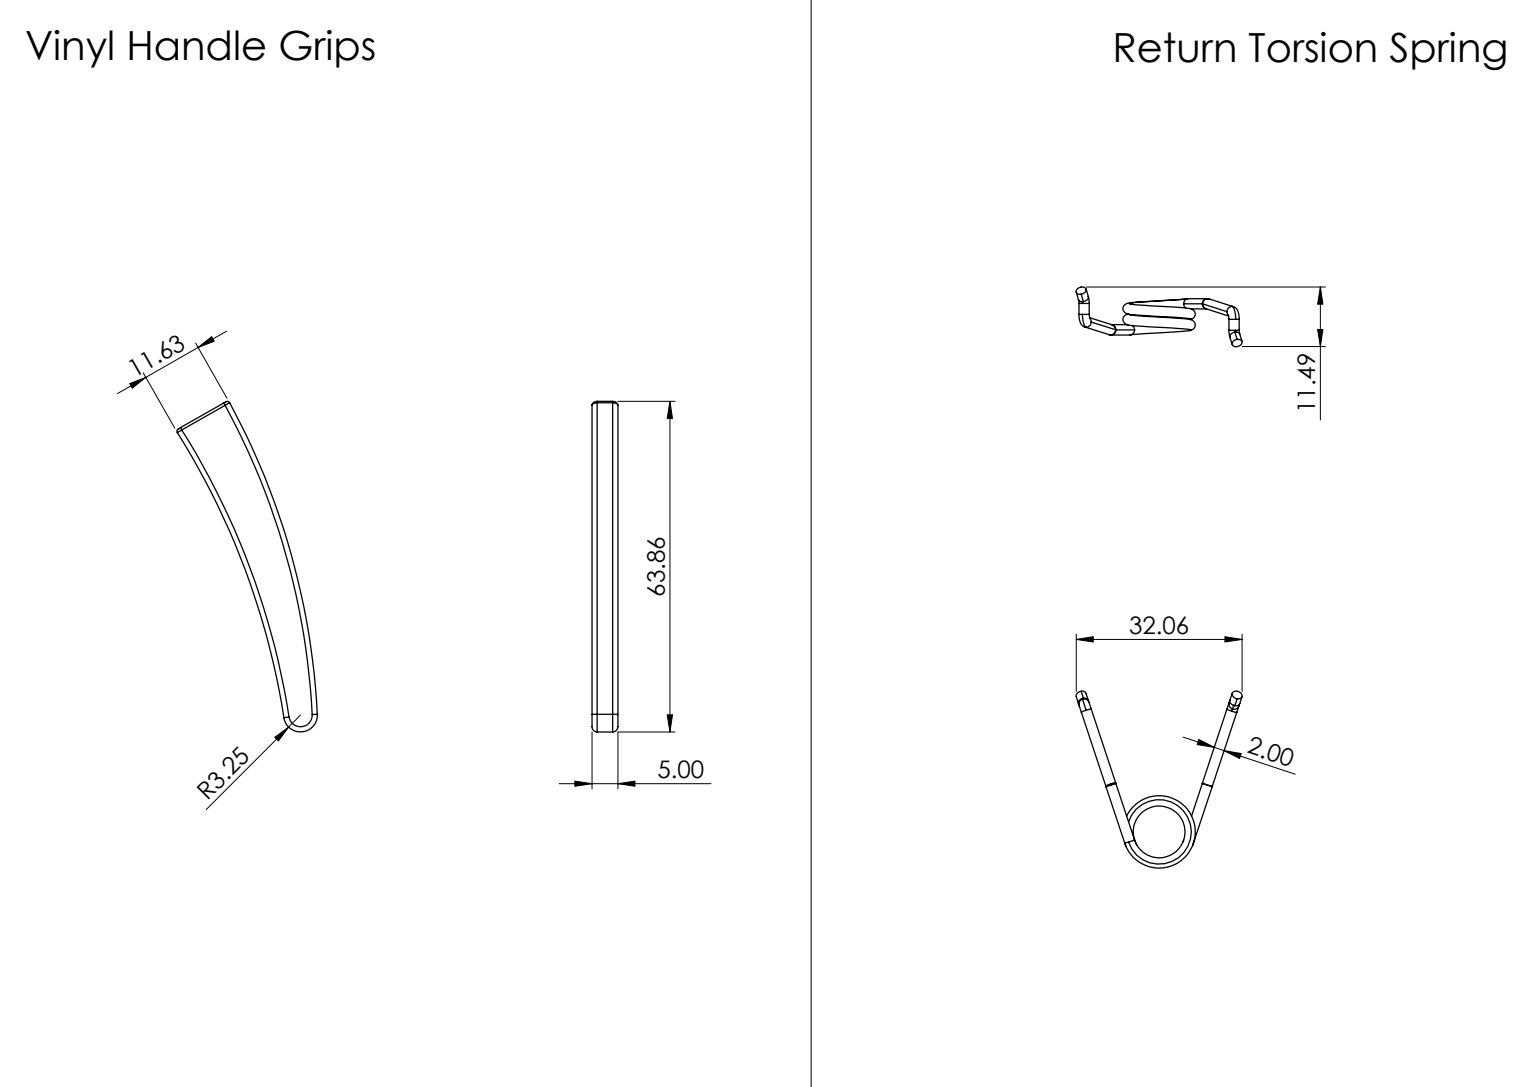
ISO-10303-21;
HEADER;
FILE_DESCRIPTION (('STEP AP214'),
    '1' );
FILE_NAME ('Vinyl Handle Grips.step',
    '2026-10-09T15:01:35',
    ( '' ),
    ( '' ),
    'SwSTEP 2.0',
    'SolidWorks 2026',
    '' );
FILE_SCHEMA (( 'AUTOMOTIVE_DESIGN' ));
ENDSEC;

DATA;
#1=ORIENTED_EDGE ( 'NONE', *, *, #451, .F. ) ;
#30=CARTESIAN_POINT ( 'NONE',  ( 27.63595919327375938, -34.25856858997740062, -0.5081525913518375459 ) ) ;
#33=ORIENTED_EDGE ( 'NONE', *, *, #2628, .F. ) ;
#46=ORIENTED_EDGE ( 'NONE', *, *, #4272, .T. ) ;
#49=DIRECTION ( 'NONE',  ( 5.715354789845005112E-18, 9.999836672264339449E-16, -1.000000000000000000 ) ) ;
#51=SURFACE_STYLE_USAGE ( .BOTH. , #5819 ) ;
#52=DIRECTION ( 'NONE',  ( 0.000000000000000000, -1.000000000000000000, -9.973300763855647239E-16 ) ) ;
#60=CARTESIAN_POINT ( 'NONE',  ( 17.88843813672053074, -40.41242482140540204, -4.025211077939831437E-14 ) ) ;
#61=DIRECTION ( 'NONE',  ( -0.9999836672264333925, 0.005715354789844476896, 0.000000000000000000 ) ) ;
#69=CARTESIAN_POINT ( 'NONE',  ( 18.49916120972752154, -39.46430250869199341, 3.499999999999960476 ) ) ;
#72=CARTESIAN_POINT ( 'NONE',  ( 26.87031364676133194, -34.69479876584122024, -0.5000000000000345279 ) ) ;
#83=LINE ( 'NONE', #2969, #2404 ) ;
#84=EDGE_CURVE ( 'NONE', #5434, #6822, #3844, .T. ) ;
#91=CARTESIAN_POINT ( 'NONE',  ( 18.31438873653245381, -40.15745658308031807, 3.873766277856072193 ) ) ;
#93=FACE_OUTER_BOUND ( 'NONE', #5404, .T. ) ;
#107=CARTESIAN_POINT ( 'NONE',  ( 27.99155020439382469, -34.64269665048638558, -3.446982116472166490E-14 ) ) ;
#131=ORIENTED_EDGE ( 'NONE', *, *, #84, .F. ) ;
#136=CARTESIAN_POINT ( 'NONE',  ( 27.99155020439386377, -34.64269665048637137, -4.257530847521587323E-14 ) ) ;
#140=EDGE_CURVE ( 'NONE', #6822, #6113, #1025, .T. ) ;
#166=DIRECTION ( 'NONE',  ( 5.715354789845005112E-18, 9.999836672264339449E-16, -1.000000000000000000 ) ) ;
#169=CIRCLE ( 'NONE', #2691, 147.0000000000000000 ) ;
#183=ORIENTED_EDGE ( 'NONE', *, *, #2628, .T. ) ;
#185=( LENGTH_UNIT ( ) NAMED_UNIT ( * ) SI_UNIT ( .MILLI., .METRE. ) );
#202=CYLINDRICAL_SURFACE ( 'NONE', #2445, 0.5000000000000022204 ) ;
#227=DIRECTION ( 'NONE',  ( 5.715354789845004342E-18, 9.999836672264337477E-16, -1.000000000000000000 ) ) ;
#234=TOROIDAL_SURFACE ( 'NONE', #5408, 140.0000000000000000, 1.000000000000000000 ) ;
#235=EDGE_CURVE ( 'NONE', #5505, #4310, #421, .T. ) ;
#237=CARTESIAN_POINT ( 'NONE',  ( 18.49916120972751088, -39.46430250869199341, -0.5000000000000393019 ) ) ;
#245=CARTESIAN_POINT ( 'NONE',  ( -105.7473861751082040, -118.0666774205683822, 2.999999999999881428 ) ) ;
#253=EDGE_CURVE ( 'NONE', #4908, #2830, #5444, .T. ) ;
#261=EDGE_CURVE ( 'NONE', #1236, #2830, #5625, .T. ) ;
#274=UNCERTAINTY_MEASURE_WITH_UNIT (LENGTH_MEASURE( 1.000000000000000082E-05 ), #185, 'distance_accuracy_value', 'NONE');
#275=AXIS2_PLACEMENT_3D ( 'NONE', #245, #7168, #3592 ) ;
#294=ORIENTED_EDGE ( 'NONE', *, *, #1501, .T. ) ;
#298=CIRCLE ( 'NONE', #3775, 145.9999999999999716 ) ;
#313=CARTESIAN_POINT ( 'NONE',  ( 27.55235279947361349, -34.88166451341158592, 3.999999999999965361 ) ) ;
#318=CARTESIAN_POINT ( 'NONE',  ( -95.86211798318534250, -102.0316339954322018, 3.999999999999897859 ) ) ;
#344=CARTESIAN_POINT ( 'NONE',  ( 18.49916120972752509, -39.46430250869199341, 3.499999999999960476 ) ) ;
#349=FACE_OUTER_BOUND ( 'NONE', #6871, .T. ) ;
#360=FACE_OUTER_BOUND ( 'NONE', #2389, .T. ) ;
#368=DIRECTION ( 'NONE',  ( 5.715354789845005112E-18, 9.999836672264339449E-16, -1.000000000000000000 ) ) ;
#370=DIRECTION ( 'NONE',  ( -0.9999836672264335036, 0.005715354789845008589, 0.000000000000000000 ) ) ;
#372=ORIENTED_EDGE ( 'NONE', *, *, #5459, .F. ) ;
#375=CARTESIAN_POINT ( 'NONE',  ( 39.48483786921892857, -95.33781693134928048, 3.999999999999904521 ) ) ;
#386=CARTESIAN_POINT ( 'NONE',  ( -105.7473861751082040, -118.0666774205683822, 2.999999999999881428 ) ) ;
#387=CARTESIAN_POINT ( 'NONE',  ( -95.86211798318534250, -102.0316339954322018, 2.999999999999897859 ) ) ;
#391=AXIS2_PLACEMENT_3D ( 'NONE', #5186, #5641, #2797 ) ;
#393=EDGE_CURVE ( 'NONE', #1414, #6322, #2060, .T. ) ;
#401=CARTESIAN_POINT ( 'NONE',  ( 27.74785680215192940, -34.19481439742430240, 3.132117371547133100 ) ) ;
#403=ORIENTED_EDGE ( 'NONE', *, *, #803, .T. ) ;
#407=AXIS2_PLACEMENT_3D ( 'NONE', #1418, #3070, #5386 ) ;
#420=VERTEX_POINT ( 'NONE', #6767 ) ;
#421=LINE ( 'NONE', #2456, #6291 ) ;
#445=EDGE_LOOP ( 'NONE', ( #6799, #6289, #2155, #183 ) ) ;
#446=ORIENTED_EDGE ( 'NONE', *, *, #1818, .F. ) ;
#450=CARTESIAN_POINT ( 'NONE',  ( 41.70778007397900211, -94.98992620957551480, 2.999999999999905409 ) ) ;
#451=EDGE_CURVE ( 'NONE', #5505, #7068, #7351, .T. ) ;
#453=LINE ( 'NONE', #485, #6901 ) ;
#456=CARTESIAN_POINT ( 'NONE',  ( -109.1076725891878567, -112.1689003517234227, -1.127570259384924611E-13 ) ) ;
#460=ORIENTED_EDGE ( 'NONE', *, *, #4272, .F. ) ;
#462=CARTESIAN_POINT ( 'NONE',  ( 18.23198843067283548, -39.61652546476334180, 3.399839610809888946 ) ) ;
#463=DIRECTION ( 'NONE',  ( 0.9986925448795958005, 0.05111947575940636868, 0.000000000000000000 ) ) ;
#466=CARTESIAN_POINT ( 'NONE',  ( 27.55235279947335414, -34.88166451341171381, -3.471129529363089628E-14 ) ) ;
#471=CARTESIAN_POINT ( 'NONE',  ( 18.47982041150265431, -39.47532202006953383, -3.946495907847236140E-14 ) ) ;
#474=CARTESIAN_POINT ( 'NONE',  ( 18.06432739836633061, -39.71205113188396041, -3.955074325938771262E-14 ) ) ;
#481=CARTESIAN_POINT ( 'NONE',  ( -105.7473861751082040, -118.0666774205683822, -1.186117176699141851E-13 ) ) ;
#485=CARTESIAN_POINT ( 'NONE',  ( 18.06432739836633061, -39.71205113188396041, 3.999999999999960032 ) ) ;
#502=CARTESIAN_POINT ( 'NONE',  ( 18.74668230531433721, -39.89873697698325117, 3.999999999999960032 ) ) ;
#515=CARTESIAN_POINT ( 'NONE',  ( 18.38437304540687833, -39.52970360889655410, -0.5000000000000393019 ) ) ;
#527=AXIS2_PLACEMENT_3D ( 'NONE', #7403, #2247, #4554 ) ;
#530=DIRECTION ( 'NONE',  ( 0.000000000000000000, -1.000000000000000000, -8.673617379884027583E-16 ) ) ;
#531=DIRECTION ( 'NONE',  ( -0.9999836672264333925, 0.005715354789843017994, -1.984263399433601008E-30 ) ) ;
#533=LINE ( 'NONE', #2887, #6913 ) ;
#546=ORIENTED_EDGE ( 'NONE', *, *, #3188, .T. ) ;
#555=VERTEX_POINT ( 'NONE', #5918 ) ;
#556=B_SPLINE_CURVE_WITH_KNOTS ( 'NONE', 3,
 ( #5245, #2849, #6332, #5736, #1652, #5167, #596, #5949 ),
 .UNSPECIFIED., .F., .F.,
 ( 4, 2, 2, 4 ),
 ( 7.023086426956682172E-18, 0.0003905485738067056029, 0.0007810971476134041585, 0.001562194295226800728 ),
 .UNSPECIFIED. ) ;
#584=CARTESIAN_POINT ( 'NONE',  ( 18.49916120972750377, -39.46430250869199341, -0.5000000000000393019 ) ) ;
#592=CARTESIAN_POINT ( 'NONE',  ( 27.24990648202821575, -34.47852395037432416, -0.2518834531394323339 ) ) ;
#596=CARTESIAN_POINT ( 'NONE',  ( 27.99155020439387798, -34.64269665048637137, -0.2641155699549361247 ) ) ;
#612=CARTESIAN_POINT ( 'NONE',  ( 17.98171507014359349, -40.35658427893240230, 3.523056311642938088 ) ) ;
#618=CARTESIAN_POINT ( 'NONE',  ( 27.57050386326208979, -34.29586207421746735, 3.619543086858307390 ) ) ;
#626=CARTESIAN_POINT ( 'NONE',  ( 18.11162751801429849, -39.68510166472335499, 3.261603458983328263 ) ) ;
#631=CARTESIAN_POINT ( 'NONE',  ( 27.88111011609792556, -34.70420074580282943, -0.5037669066447876265 ) ) ;
#637=TOROIDAL_SURFACE ( 'NONE', #2433, 2.249999999999964917, 1.000000000000000000 ) ;
#647=AXIS2_PLACEMENT_3D ( 'NONE', #7275, #6601, #6098 ) ;
#673=CARTESIAN_POINT ( 'NONE',  ( 18.06432739836606771, -39.71205113188410962, 2.999999999999960476 ) ) ;
#676=EDGE_CURVE ( 'NONE', #888, #2009, #2043, .T. ) ;
#706=ADVANCED_FACE ( 'NONE', ( #360 ), #1383, .T. ) ;
#709=AXIS2_PLACEMENT_3D ( 'NONE', #6443, #2440, #1841 ) ;
#717=DIRECTION ( 'NONE',  ( 5.715354789845005112E-18, 9.999836672264339449E-16, -1.000000000000000000 ) ) ;
#718=CARTESIAN_POINT ( 'NONE',  ( 39.48483786921892857, -95.33781693134928048, 3.999999999999904521 ) ) ;
#721=CARTESIAN_POINT ( 'NONE',  ( 18.11927033577788393, -39.68074713310974744, -0.2519513543403087419 ) ) ;
#731=CARTESIAN_POINT ( 'NONE',  ( 26.87807528571524074, -34.69037653529182563, 2.999999999999965361 ) ) ;
#745=CIRCLE ( 'NONE', #1355, 147.0000000000000000 ) ;
#750=EDGE_CURVE ( 'NONE', #6928, #6113, #6639, .T. ) ;
#751=AXIS2_PLACEMENT_3D ( 'NONE', #5959, #3597, #6467 ) ;
#762=CARTESIAN_POINT ( 'NONE',  ( -95.86211798318534250, -102.0316339954322018, 3.999999999999897859 ) ) ;
#763=CARTESIAN_POINT ( 'NONE',  ( 17.88843813772660596, -40.41242482300715011, -0.1308508315819079393 ) ) ;
#765=CIRCLE ( 'NONE', #6539, 0.5000000000000004441 ) ;
#767=AXIS2_PLACEMENT_3D ( 'NONE', #871, #3769, #5908 ) ;
#774=AXIS2_PLACEMENT_3D ( 'NONE', #1957, #4270, #4224 ) ;
#802=EDGE_CURVE ( 'NONE', #7250, #6854, #6673, .T. ) ;
#803=EDGE_CURVE ( 'NONE', #5496, #7250, #1244, .T. ) ;
#816=DIRECTION ( 'NONE',  ( -5.715354789845005112E-18, -9.999836672264339449E-16, 1.000000000000000000 ) ) ;
#818=CARTESIAN_POINT ( 'NONE',  ( 27.11783474234813340, -35.12923323413248511, 3.499999999999964917 ) ) ;
#819=DIRECTION ( 'NONE',  ( -0.9999836672264335036, 0.005715354789845008589, 0.000000000000000000 ) ) ;
#824=CYLINDRICAL_SURFACE ( 'NONE', #5814, 2.249999999999962252 ) ;
#851=ORIENTED_EDGE ( 'NONE', *, *, #4724, .T. ) ;
#863=STYLED_ITEM ( 'NONE', ( #5858 ), #2394 ) ;
#869=TOROIDAL_SURFACE ( 'NONE', #275, 147.0000000000000000, 1.000000000000000000 ) ;
#871=CARTESIAN_POINT ( 'NONE',  ( 27.55235279947361349, -34.88166451341158592, 3.999999999999965361 ) ) ;
#884=CARTESIAN_POINT ( 'NONE',  ( 17.88843813672055916, -40.41242482140537362, 3.999999999999959144 ) ) ;
#888=VERTEX_POINT ( 'NONE', #5085 ) ;
#896=DIRECTION ( 'NONE',  ( 5.715354789845005112E-18, 9.999836672264339449E-16, -1.000000000000000000 ) ) ;
#911=FACE_OUTER_BOUND ( 'NONE', #4195, .T. ) ;
#927=ORIENTED_EDGE ( 'NONE', *, *, #5460, .F. ) ;
#932=DIRECTION ( 'NONE',  ( 5.715354789845005112E-18, 9.999836672264339449E-16, -1.000000000000000000 ) ) ;
#936=VERTEX_POINT ( 'NONE', #107 ) ;
#939=LINE ( 'NONE', #456, #5214 ) ;
#941=DIRECTION ( 'NONE',  ( 5.715354789845005112E-18, 9.999836672264339449E-16, -1.000000000000000000 ) ) ;
#958=CARTESIAN_POINT ( 'NONE',  ( 27.99155020439384955, -34.64269665048638558, 2.999999999999965361 ) ) ;
#968=FACE_OUTER_BOUND ( 'NONE', #3719, .T. ) ;
#989=( GEOMETRIC_REPRESENTATION_CONTEXT ( 3 ) GLOBAL_UNCERTAINTY_ASSIGNED_CONTEXT ( ( #274 ) ) GLOBAL_UNIT_ASSIGNED_CONTEXT ( ( #185, #5991, #3638 ) ) REPRESENTATION_CONTEXT ( 'NONE', 'WORKASPACE' ) );
#1002=ORIENTED_EDGE ( 'NONE', *, *, #7088, .T. ) ;
#1004=ORIENTED_EDGE ( 'NONE', *, *, #7088, .F. ) ;
#1006=CIRCLE ( 'NONE', #647, 147.0000000000000000 ) ;
#1014=EDGE_LOOP ( 'NONE', ( #403, #1276, #2986, #6808 ) ) ;
#1021=CARTESIAN_POINT ( 'NONE',  ( 27.88123484459569568, -34.70413128614676168, 3.503735202131379900 ) ) ;
#1024=ORIENTED_EDGE ( 'NONE', *, *, #261, .T. ) ;
#1025=B_SPLINE_CURVE_WITH_KNOTS ( 'NONE', 3,
 ( #4575, #3398, #2302, #91, #1665, #612, #4005, #4077 ),
 .UNSPECIFIED., .F., .F.,
 ( 4, 2, 2, 4 ),
 ( 0.000000000000000000, 0.0003905813100143790020, 0.0007811626200287574619, 0.001562325240057513189 ),
 .UNSPECIFIED. ) ;
#1027=CARTESIAN_POINT ( 'NONE',  ( 17.79267347262679522, -39.86682724249966014, 3.626282107859409187 ) ) ;
#1032=DIRECTION ( 'NONE',  ( -3.391455187862681927E-16, -1.191495097990696953E-15, 1.000000000000000000 ) ) ;
#1055=DIRECTION ( 'NONE',  ( -3.391455187862681927E-16, -1.191495097990696953E-15, 1.000000000000000000 ) ) ;
#1059=CARTESIAN_POINT ( 'NONE',  ( 27.81639631407590585, -34.74023945865230445, 3.614623298852130517 ) ) ;
#1063=CARTESIAN_POINT ( 'NONE',  ( 18.31450325791856315, -40.15738803827605352, 3.873838653338203208 ) ) ;
#1074=TOROIDAL_SURFACE ( 'NONE', #2746, 140.0000000000000000, 1.000000000000000000 ) ;
#1081=AXIS2_PLACEMENT_3D ( 'NONE', #1259, #3654, #5970 ) ;
#1087=DIRECTION ( 'NONE',  ( 5.715354789845005112E-18, 9.999836672264339449E-16, -1.000000000000000000 ) ) ;
#1092=FACE_OUTER_BOUND ( 'NONE', #2421, .T. ) ;
#1097=CARTESIAN_POINT ( 'NONE',  ( -108.8601514936008385, -112.6033348200152773, 3.499999999999886757 ) ) ;
#1098=DIRECTION ( 'NONE',  ( -5.715354789845005112E-18, -9.999836672264339449E-16, 1.000000000000000000 ) ) ;
#1101=ORIENTED_EDGE ( 'NONE', *, *, #3974, .T. ) ;
#1117=ORIENTED_EDGE ( 'NONE', *, *, #1901, .T. ) ;
#1123=AXIS2_PLACEMENT_3D ( 'NONE', #4973, #5514, #2057 ) ;
#1131=EDGE_LOOP ( 'NONE', ( #4538, #294, #3018, #5684 ) ) ;
#1140=VECTOR ( 'NONE', #4420, 1000.000000000000000 ) ;
#1142=LINE ( 'NONE', #2372, #5672 ) ;
#1159=DIRECTION ( 'NONE',  ( -2.925622616928933849E-16, -1.164954066665946421E-15, 1.000000000000000000 ) ) ;
#1166=CYLINDRICAL_SURFACE ( 'NONE', #527, 0.5000000000000004441 ) ;
#1168=CARTESIAN_POINT ( 'NONE',  ( 27.55792021817859805, -34.88417811465595264, -0.8737629652053834350 ) ) ;
#1177=CARTESIAN_POINT ( 'NONE',  ( -105.7473861751082040, -118.0666774205683822, 3.999999999999881428 ) ) ;
#1181=CARTESIAN_POINT ( 'NONE',  ( 18.44231076305980466, -39.49669331989797172, 3.499999956044343552 ) ) ;
#1182=EDGE_CURVE ( 'NONE', #6822, #2064, #5580, .T. ) ;
#1189=DIRECTION ( 'NONE',  ( -0.9879743132267160277, -0.1546180985661085583, 0.000000000000000000 ) ) ;
#1197=ORIENTED_EDGE ( 'NONE', *, *, #7043, .T. ) ;
#1198=VERTEX_POINT ( 'NONE', #6993 ) ;
#1203=FACE_OUTER_BOUND ( 'NONE', #5268, .T. ) ;
#1231=VERTEX_POINT ( 'NONE', #2096 ) ;
#1236=VERTEX_POINT ( 'NONE', #2622 ) ;
#1244=CIRCLE ( 'NONE', #391, 0.5000000000000022204 ) ;
#1259=CARTESIAN_POINT ( 'NONE',  ( -95.86211798318534250, -102.0316339954322018, 2.999999999999897859 ) ) ;
#1264=APPLICATION_CONTEXT ( 'automotive_design' ) ;
#1268=CARTESIAN_POINT ( 'NONE',  ( 17.99687608643026593, -40.34751144403527690, -0.5039026972369210489 ) ) ;
#1276=ORIENTED_EDGE ( 'NONE', *, *, #3188, .F. ) ;
#1283=CARTESIAN_POINT ( 'NONE',  ( 27.30483170388658110, -34.44723004512043474, -3.833102624698575208E-14 ) ) ;
#1297=DIRECTION ( 'NONE',  ( -0.4950421911735689018, 0.8688689365825386091, 0.000000000000000000 ) ) ;
#1306=ORIENTED_EDGE ( 'NONE', *, *, #4864, .T. ) ;
#1309=DIRECTION ( 'NONE',  ( -0.9999836672264335036, 0.005715354789845041548, 0.000000000000000000 ) ) ;
#1312=ORIENTED_EDGE ( 'NONE', *, *, #7327, .F. ) ;
#1316=DIRECTION ( 'NONE',  ( -0.9879743132267160277, -0.1546180985661085583, -1.602621969470663276E-16 ) ) ;
#1321=ADVANCED_FACE ( 'NONE', ( #5573 ), #6181, .T. ) ;
#1332=CARTESIAN_POINT ( 'NONE',  ( 18.06432743677800445, -39.71205110999872545, -0.06542542002766411902 ) ) ;
#1354=VERTEX_POINT ( 'NONE', #2703 ) ;
#1355=AXIS2_PLACEMENT_3D ( 'NONE', #1984, #816, #5967 ) ;
#1359=SURFACE_STYLE_FILL_AREA ( #4219 ) ;
#1370=DIRECTION ( 'NONE',  ( -0.9999836672264333925, 0.005715354789844984303, 0.000000000000000000 ) ) ;
#1379=CIRCLE ( 'NONE', #7379, 1.000000000000001998 ) ;
#1383=( BOUNDED_SURFACE ( )  B_SPLINE_SURFACE ( 3, 2, ( 
 ( #4396, #6133, #958 ),
 ( #5566, #401, #2694 ),
 ( #3894, #5069, #5115 ),
 ( #4013, #6208, #6828 ),
 ( #7352, #618, #7395 ),
 ( #6352, #6867, #1713 ),
 ( #3477, #4546, #5152 ),
 ( #1756, #4052, #7313 ),
 ( #6278, #4512, #5676 ),
 ( #3928, #4627, #6318 ) ),
 .UNSPECIFIED., .F., .F., .F. ) 
 B_SPLINE_SURFACE_WITH_KNOTS ( ( 4, 2, 2, 2, 4 ),
 ( 3, 3 ),
 ( -2.981555974335137194E-18, 0.0001952886961233724105, 0.0003905773922467478025, 0.0005858660883701231675, 0.0007811547844934985324 ),
 ( 0.000000000000000000, 1.000000000000000000 ),
 .UNSPECIFIED. ) 
 GEOMETRIC_REPRESENTATION_ITEM ( )  RATIONAL_B_SPLINE_SURFACE ( (
 ( 1.000000000000000000, 0.7001503461741274137, 1.000000000000000000),
 ( 1.000000000000000000, 0.7001491056773789801, 1.000000000000000000),
 ( 1.000000000000000000, 0.7003313827919757095, 1.000000000000000000),
 ( 1.000000000000000000, 0.7010298770397929147, 1.000000000000000000),
 ( 1.000000000000000000, 0.7015467090662059757, 1.000000000000000000),
 ( 1.000000000000000000, 0.7028299121717020981, 1.000000000000000000),
 ( 1.000000000000000000, 0.7036054228162287316, 1.000000000000000000),
 ( 1.000000000000000000, 0.7052774926288423174, 1.000000000000000000),
 ( 1.000000000000000000, 0.7061929979163744653, 1.000000000000000000),
 ( 1.000000000000000000, 0.7071067811865477948, 1.000000000000000000) ) ) 
 REPRESENTATION_ITEM ( '' )  SURFACE ( )  );
#1408=ORIENTED_EDGE ( 'NONE', *, *, #7380, .T. ) ;
#1414=VERTEX_POINT ( 'NONE', #6324 ) ;
#1418=CARTESIAN_POINT ( 'NONE',  ( -105.7473861751082040, -118.0666774205683822, 3.999999999999881428 ) ) ;
#1430=LINE ( 'NONE', #3720, #3512 ) ;
#1443=DIRECTION ( 'NONE',  ( 5.715354789845005112E-18, 9.999836672264339449E-16, -1.000000000000000000 ) ) ;
#1478=AXIS2_PLACEMENT_3D ( 'NONE', #481, #368, #6653 ) ;
#1488=AXIS2_PLACEMENT_3D ( 'NONE', #3820, #1087, #370 ) ;
#1501=EDGE_CURVE ( 'NONE', #6491, #1414, #1839, .T. ) ;
#1534=FACE_OUTER_BOUND ( 'NONE', #5497, .T. ) ;
#1535=DIRECTION ( 'NONE',  ( 5.715354789845005112E-18, 9.999836672264339449E-16, -1.000000000000000000 ) ) ;
#1539=EDGE_CURVE ( 'NONE', #6928, #1231, #5117, .T. ) ;
#1549=DIRECTION ( 'NONE',  ( -5.715354789845005112E-18, -9.999836672264339449E-16, 1.000000000000000000 ) ) ;
#1565=ORIENTED_EDGE ( 'NONE', *, *, #253, .T. ) ;
#1596=ORIENTED_EDGE ( 'NONE', *, *, #3604, .F. ) ;
#1604=LINE ( 'NONE', #884, #4615 ) ;
#1625=CARTESIAN_POINT ( 'NONE',  ( 18.38544986348231447, -39.52909008669877977, 3.487024505045074996 ) ) ;
#1629=CARTESIAN_POINT ( 'NONE',  ( 18.74668230531428748, -39.89873697698326538, -1.000000000000039968 ) ) ;
#1652=CARTESIAN_POINT ( 'NONE',  ( 27.65482637540493016, -34.83021424519443343, -0.7995430095508657686 ) ) ;
#1655=CARTESIAN_POINT ( 'NONE',  ( 27.57479190627129384, -34.87478370679277617, 3.891341692651370199 ) ) ;
#1665=CARTESIAN_POINT ( 'NONE',  ( 18.21922820888615036, -40.21441497322944514, 3.799573870912058116 ) ) ;
#1681=ADVANCED_FACE ( 'NONE', ( #7059 ), #2390, .F. ) ;
#1700=CARTESIAN_POINT ( 'NONE',  ( 18.06097555607235705, -40.30914097186184364, 3.615364355270606289 ) ) ;
#1705=ORIENTED_EDGE ( 'NONE', *, *, #5741, .T. ) ;
#1713=CARTESIAN_POINT ( 'NONE',  ( 27.65530182349729671, -34.82994948188742512, 3.799124122364484712 ) ) ;
#1720=VECTOR ( 'NONE', #6644, 1000.000000000000000 ) ;
#1721=PRODUCT_CONTEXT ( 'NONE', #1264, 'mechanical' ) ;
#1727=CARTESIAN_POINT ( 'NONE',  ( 27.11783474234811564, -35.12923323413249221, -1.000000000000034861 ) ) ;
#1744=AXIS2_PLACEMENT_3D ( 'NONE', #762, #1916, #4877 ) ;
#1756=CARTESIAN_POINT ( 'NONE',  ( 26.98470030103655404, -34.62962642788639300, 3.486735179637458604 ) ) ;
#1768=ORIENTED_EDGE ( 'NONE', *, *, #393, .F. ) ;
#1778=DIRECTION ( 'NONE',  ( 5.715354789845004342E-18, 9.999836672264337477E-16, -1.000000000000000000 ) ) ;
#1779=CARTESIAN_POINT ( 'NONE',  ( 43.95483829995806957, -94.87490738911687060, 2.999999999999905409 ) ) ;
#1786=DIRECTION ( 'NONE',  ( -0.1546180985661130547, 0.9879743132267154726, 9.870744795757317374E-16 ) ) ;
#1798=CARTESIAN_POINT ( 'NONE',  ( 27.65480120734329006, -34.83022826066387267, -0.7995651912284664764 ) ) ;
#1803=ADVANCED_BREP_SHAPE_REPRESENTATION ( '', ( #2394, #751 ), #989 ) ;
#1816=ORIENTED_EDGE ( 'NONE', *, *, #3604, .T. ) ;
#1818=EDGE_CURVE ( 'NONE', #2009, #6491, #1006, .T. ) ;
#1824=ORIENTED_EDGE ( 'NONE', *, *, #5459, .T. ) ;
#1839=CIRCLE ( 'NONE', #4008, 2.249999999999962252 ) ;
#1841=DIRECTION ( 'NONE',  ( -0.9999836672264332815, 0.005715354789842956411, 0.000000000000000000 ) ) ;
#1844=AXIS2_PLACEMENT_3D ( 'NONE', #2492, #166, #1370 ) ;
#1847=AXIS2_PLACEMENT_3D ( 'NONE', #7148, #227, #2518 ) ;
#1854=ORIENTED_EDGE ( 'NONE', *, *, #6843, .F. ) ;
#1885=CYLINDRICAL_SURFACE ( 'NONE', #2212, 0.5000000000000004441 ) ;
#1886=CARTESIAN_POINT ( 'NONE',  ( 17.61082888335783991, -39.97043405836763696, -0.1337947118489001552 ) ) ;
#1901=EDGE_CURVE ( 'NONE', #3586, #5496, #6981, .T. ) ;
#1916=DIRECTION ( 'NONE',  ( -5.715354789845005112E-18, -9.999836672264339449E-16, 1.000000000000000000 ) ) ;
#1917=FACE_OUTER_BOUND ( 'NONE', #3479, .T. ) ;
#1957=CARTESIAN_POINT ( 'NONE',  ( 41.70778007397900211, -94.98992620957551480, -1.000000000000094591 ) ) ;
#1958=CARTESIAN_POINT ( 'NONE',  ( 18.74668230531429458, -39.89873697698326538, -1.000000000000039746 ) ) ;
#1984=CARTESIAN_POINT ( 'NONE',  ( -105.7473861751082040, -118.0666774205683822, -1.000000000000118794 ) ) ;
#2009=VERTEX_POINT ( 'NONE', #471 ) ;
#2016=ORIENTED_EDGE ( 'NONE', *, *, #1182, .T. ) ;
#2034=ORIENTED_EDGE ( 'NONE', *, *, #802, .F. ) ;
#2036=EDGE_CURVE ( 'NONE', #420, #7068, #3939, .T. ) ;
#2043=LINE ( 'NONE', #4352, #1720 ) ;
#2048=ORIENTED_EDGE ( 'NONE', *, *, #3336, .T. ) ;
#2057=DIRECTION ( 'NONE',  ( -0.9999836672264333925, 0.005715354789844970425, 0.000000000000000000 ) ) ;
#2060=CIRCLE ( 'NONE', #5815, 140.0000000000000000 ) ;
#2064=VERTEX_POINT ( 'NONE', #718 ) ;
#2068=CARTESIAN_POINT ( 'NONE',  ( 41.70778007397900211, -94.98992620957551480, 3.999999999999905409 ) ) ;
#2086=ADVANCED_FACE ( 'NONE', ( #3800 ), #7117, .T. ) ;
#2087=ADVANCED_FACE ( 'NONE', ( #911 ), #824, .F. ) ;
#2091=ORIENTED_EDGE ( 'NONE', *, *, #5846, .F. ) ;
#2096=CARTESIAN_POINT ( 'NONE',  ( 18.49916120972752154, -39.46430250869199341, 3.499999999999960476 ) ) ;
#2100=EDGE_LOOP ( 'NONE', ( #446, #5456, #4019, #5209 ) ) ;
#2107=DIRECTION ( 'NONE',  ( -0.8688689365825387201, -0.4950421911735688463, -4.999999999999992500E-16 ) ) ;
#2150=APPLICATION_CONTEXT ( 'automotive_design' ) ;
#2155=ORIENTED_EDGE ( 'NONE', *, *, #4864, .F. ) ;
#2167=EDGE_CURVE ( 'NONE', #3782, #1414, #1430, .T. ) ;
#2177=AXIS2_PLACEMENT_3D ( 'NONE', #6222, #1055, #530 ) ;
#2184=CIRCLE ( 'NONE', #5086, 2.249999999999962252 ) ;
#2194=ADVANCED_FACE ( 'NONE', ( #3198 ), #4514, .T. ) ;
#2203=EDGE_LOOP ( 'NONE', ( #1705, #5259, #2016, #2577 ) ) ;
#2212=AXIS2_PLACEMENT_3D ( 'NONE', #313, #6561, #6592 ) ;
#2220=CARTESIAN_POINT ( 'NONE',  ( -95.86211798318534250, -102.0316339954322018, -1.025655255171287195E-13 ) ) ;
#2226=CARTESIAN_POINT ( 'NONE',  ( 18.06432739836606771, -39.71205113188410962, 2.999999999999959144 ) ) ;
#2228=CARTESIAN_POINT ( 'NONE',  ( 27.55235279947361349, -34.38166451341171381, -3.421263025543810879E-14 ) ) ;
#2237=LINE ( 'NONE', #4510, #2564 ) ;
#2243=VERTEX_POINT ( 'NONE', #5629 ) ;
#2246=ORIENTED_EDGE ( 'NONE', *, *, #6154, .F. ) ;
#2247=DIRECTION ( 'NONE',  ( 5.715354789845005112E-18, 9.999836672264339449E-16, -1.000000000000000000 ) ) ;
#2249=PLANE ( 'NONE',  #2332 ) ;
#2251=ORIENTED_EDGE ( 'NONE', *, *, #7295, .T. ) ;
#2252=ORIENTED_EDGE ( 'NONE', *, *, #3180, .F. ) ;
#2268=CARTESIAN_POINT ( 'NONE',  ( 18.74668230531428748, -39.89873697698326538, -1.000000000000039968 ) ) ;
#2276=VERTEX_POINT ( 'NONE', #3390 ) ;
#2283=CARTESIAN_POINT ( 'NONE',  ( 27.23210503485723777, -35.06560599256804522, -1.000000000000034861 ) ) ;
#2302=CARTESIAN_POINT ( 'NONE',  ( 18.52216156081266618, -40.03310245541522505, 3.974029017541355291 ) ) ;
#2304=CARTESIAN_POINT ( 'NONE',  ( 39.48483786921892857, -95.33781693134928048, 2.999999999999904521 ) ) ;
#2326=CARTESIAN_POINT ( 'NONE',  ( 27.29329919813223526, -34.45380074488651445, -0.1316498810018032206 ) ) ;
#2332=AXIS2_PLACEMENT_3D ( 'NONE', #5040, #3221, #1535 ) ;
#2346=( LENGTH_UNIT ( ) NAMED_UNIT ( * ) SI_UNIT ( .MILLI., .METRE. ) );
#2357=ADVANCED_FACE ( 'NONE', ( #3499 ), #6967, .T. ) ;
#2363=CARTESIAN_POINT ( 'NONE',  ( 27.96836146114586441, -34.65561064741672226, -0.2632997616376124284 ) ) ;
#2372=CARTESIAN_POINT ( 'NONE',  ( 44.95353084483765826, -94.82378791335750634, 3.999999999999905409 ) ) ;
#2377=( NAMED_UNIT ( * ) SI_UNIT ( $, .STERADIAN. ) SOLID_ANGLE_UNIT ( ) );
#2382=CARTESIAN_POINT ( 'NONE',  ( 18.05682957847944436, -39.71632305027067389, -0.8833408112552532110 ) ) ;
#2386=( BOUNDED_SURFACE ( )  B_SPLINE_SURFACE ( 3, 2, ( 
 ( #2978, #6422, #3055 ),
 ( #1332, #1886, #763 ),
 ( #3661, #5262, #5977 ),
 ( #721, #5935, #1268 ),
 ( #4798, #6482, #4834 ),
 ( #4725, #4160, #3549 ),
 ( #6452, #2382, #3581 ),
 ( #5864, #7081, #3617 ),
 ( #3689, #5896, #5398 ),
 ( #237, #7119, #1958 ) ),
 .UNSPECIFIED., .F., .F., .T. ) 
 B_SPLINE_SURFACE_WITH_KNOTS ( ( 4, 2, 2, 2, 4 ),
 ( 3, 3 ),
 ( 0.000000000000000000, 0.0001953595625521471020, 0.0003907191251042942039, 0.0005860786876564413059, 0.0007814382502085884079 ),
 ( 0.000000000000000000, 1.000000000000000000 ),
 .UNSPECIFIED. ) 
 GEOMETRIC_REPRESENTATION_ITEM ( )  RATIONAL_B_SPLINE_SURFACE ( (
 ( 1.000000000000000000, 0.6917656125192643835, 1.000000000000000000),
 ( 1.000000000000000000, 0.6917626678221141523, 1.000000000000000000),
 ( 1.000000000000000000, 0.6921708295056779869, 1.000000000000000000),
 ( 1.000000000000000000, 0.6937291441607075226, 1.000000000000000000),
 ( 1.000000000000000000, 0.6948807116037144516, 1.000000000000000000),
 ( 1.000000000000000000, 0.6977261400977853301, 1.000000000000000000),
 ( 1.000000000000000000, 0.6994400533938299747, 1.000000000000000000),
 ( 1.000000000000000000, 0.7031153542365370379, 1.000000000000000000),
 ( 1.000000000000000000, 0.7051186676678535825, 1.000000000000000000),
 ( 1.000000000000000000, 0.7071067811865472397, 1.000000000000000000) ) ) 
 REPRESENTATION_ITEM ( '' )  SURFACE ( )  );
#2388=VERTEX_POINT ( 'NONE', #5888 ) ;
#2389=EDGE_LOOP ( 'NONE', ( #3062, #6776, #1824, #6331, #3971 ) ) ;
#2390=PLANE ( 'NONE',  #4114 ) ;
#2393=CARTESIAN_POINT ( 'NONE',  ( 27.57011700825883693, -34.29608248668765214, -0.6201149797898980465 ) ) ;
#2394=MANIFOLD_SOLID_BREP ( 'Stock-MAS-689-1', #3615 ) ;
#2404=VECTOR ( 'NONE', #1098, 1000.000000000000000 ) ;
#2421=EDGE_LOOP ( 'NONE', ( #4697, #4071, #2541, #3463 ) ) ;
#2433=AXIS2_PLACEMENT_3D ( 'NONE', #4645, #7410, #531 ) ;
#2440=DIRECTION ( 'NONE',  ( 5.715354789845005112E-18, 9.999836672264339449E-16, -1.000000000000000000 ) ) ;
#2445=AXIS2_PLACEMENT_3D ( 'NONE', #5326, #2529, #1297 ) ;
#2448=CIRCLE ( 'NONE', #1488, 140.0000000000000000 ) ;
#2455=EDGE_CURVE ( 'NONE', #1198, #3782, #2184, .T. ) ;
#2456=CARTESIAN_POINT ( 'NONE',  ( 27.55235279947361349, -34.38166451341158592, 3.999999999999966249 ) ) ;
#2457=CARTESIAN_POINT ( 'NONE',  ( 18.31184849395284786, -40.14648560017537449, -3.998375596128007773E-14 ) ) ;
#2466=EDGE_CURVE ( 'NONE', #420, #5434, #6057, .T. ) ;
#2467=ORIENTED_EDGE ( 'NONE', *, *, #6733, .F. ) ;
#2492=CARTESIAN_POINT ( 'NONE',  ( -105.7473861751082040, -118.0666774205683822, 3.999999999999881428 ) ) ;
#2518=DIRECTION ( 'NONE',  ( -0.005715354789845003385, -0.9999836672264335036, -1.000000000000000472E-15 ) ) ;
#2526=CARTESIAN_POINT ( 'NONE',  ( 27.09727426766168534, -34.56548687730422387, -0.4458683620789745672 ) ) ;
#2529=DIRECTION ( 'NONE',  ( 0.8688689365825387201, 0.4950421911735688463, 4.999999999999993486E-16 ) ) ;
#2541=ORIENTED_EDGE ( 'NONE', *, *, #6003, .F. ) ;
#2550=DIRECTION ( 'NONE',  ( -5.715354789845005112E-18, -9.999836672264339449E-16, 1.000000000000000000 ) ) ;
#2553=MECHANICAL_DESIGN_GEOMETRIC_PRESENTATION_REPRESENTATION('',(#863),#3627);
#2564=VECTOR ( 'NONE', #6276, 1000.000000000000000 ) ;
#2574=CIRCLE ( 'NONE', #774, 2.249999999999962252 ) ;
#2576=DIRECTION ( 'NONE',  ( -0.9999836672264333925, 0.005715354789844970425, 0.000000000000000000 ) ) ;
#2577=ORIENTED_EDGE ( 'NONE', *, *, #3180, .T. ) ;
#2601=DIRECTION ( 'NONE',  ( -0.005715354789845003385, -0.9999836672264335036, -1.000000000000000472E-15 ) ) ;
#2604=PRODUCT_DEFINITION_CONTEXT ( 'detailed design', #2150, 'design' ) ;
#2610=ORIENTED_EDGE ( 'NONE', *, *, #2167, .F. ) ;
#2622=CARTESIAN_POINT ( 'NONE',  ( 27.30483170388656333, -34.44723004512044895, -3.427979277949995323E-14 ) ) ;
#2626=ORIENTED_EDGE ( 'NONE', *, *, #5743, .T. ) ;
#2628=EDGE_CURVE ( 'NONE', #2388, #4165, #5455, .T. ) ;
#2631=EDGE_LOOP ( 'NONE', ( #5850, #1408, #5648, #7101 ) ) ;
#2635=ADVANCED_FACE ( 'NONE', ( #7437 ), #1166, .T. ) ;
#2637=DIRECTION ( 'NONE',  ( -0.9999836672264333925, 0.005715354789844476896, 0.000000000000000000 ) ) ;
#2663=LINE ( 'NONE', #3374, #4610 ) ;
#2670=AXIS2_PLACEMENT_3D ( 'NONE', #5581, #4301, #4157 ) ;
#2678=UNCERTAINTY_MEASURE_WITH_UNIT (LENGTH_MEASURE( 1.000000000000000082E-05 ), #2346, 'distance_accuracy_value', 'NONE');
#2684=CARTESIAN_POINT ( 'NONE',  ( 27.55235279947333993, -34.88166451341173513, 2.999999999999965361 ) ) ;
#2691=AXIS2_PLACEMENT_3D ( 'NONE', #6675, #4775, #1309 ) ;
#2694=CARTESIAN_POINT ( 'NONE',  ( 27.99155020480830913, -34.64269665124812292, 3.130807245034128883 ) ) ;
#2703=CARTESIAN_POINT ( 'NONE',  ( 39.48483786921892857, -95.33781693134928048, -1.000000000000095035 ) ) ;
#2714=CARTESIAN_POINT ( 'NONE',  ( 18.74668230531430879, -39.89873697698326538, 3.499999999999960032 ) ) ;
#2733=DIRECTION ( 'NONE',  ( -5.715354789845005112E-18, -9.999836672264339449E-16, 1.000000000000000000 ) ) ;
#2741=EDGE_LOOP ( 'NONE', ( #2048, #131, #5871, #2091 ) ) ;
#2742=CARTESIAN_POINT ( 'NONE',  ( 17.91123389404125277, -40.39877837690324469, 3.263394571671051292 ) ) ;
#2746=AXIS2_PLACEMENT_3D ( 'NONE', #6413, #5317, #3544 ) ;
#2754=CARTESIAN_POINT ( 'NONE',  ( 18.27182554301009532, -39.59382808135931242, -0.4457246814534224222 ) ) ;
#2777=ADVANCED_FACE ( 'NONE', ( #4740 ), #869, .T. ) ;
#2793=VECTOR ( 'NONE', #5451, 1000.000000000000000 ) ;
#2797=DIRECTION ( 'NONE',  ( -0.4950421911735689018, 0.8688689365825386091, 0.000000000000000000 ) ) ;
#2802=ORIENTED_EDGE ( 'NONE', *, *, #6003, .T. ) ;
#2804=DIRECTION ( 'NONE',  ( -0.9999836672264333925, 0.005715354789844476896, 0.000000000000000000 ) ) ;
#2811=AXIS2_PLACEMENT_3D ( 'NONE', #4289, #5993, #6141 ) ;
#2818=EDGE_CURVE ( 'NONE', #2276, #6322, #5906, .T. ) ;
#2830=VERTEX_POINT ( 'NONE', #5951 ) ;
#2841=DIRECTION ( 'NONE',  ( -5.715354789845005112E-18, -9.999836672264339449E-16, 1.000000000000000000 ) ) ;
#2847=EDGE_LOOP ( 'NONE', ( #5275, #4432, #6575, #2467 ) ) ;
#2849=CARTESIAN_POINT ( 'NONE',  ( 27.23321219009249816, -35.06498951359424865, -1.000000000000034861 ) ) ;
#2866=CARTESIAN_POINT ( 'NONE',  ( 18.52003153382460354, -40.03437257541853711, -1.000000000000039746 ) ) ;
#2877=CARTESIAN_POINT ( 'NONE',  ( 41.70778007397900211, -94.98992620957551480, -9.475926987523308753E-14 ) ) ;
#2887=CARTESIAN_POINT ( 'NONE',  ( 17.61001731287966265, -39.97089645448942719, 3.499999999999960032 ) ) ;
#2889=CARTESIAN_POINT ( 'NONE',  ( 27.34858876736844380, -35.00074627774458946, 3.999999999999965361 ) ) ;
#2891=CARTESIAN_POINT ( 'NONE',  ( -105.7473861751082040, -118.0666774205683822, 2.999999999999881428 ) ) ;
#2905=EDGE_CURVE ( 'NONE', #6113, #3586, #1604, .T. ) ;
#2921=CARTESIAN_POINT ( 'NONE',  ( 27.34640600250860487, -35.00195951109004255, -0.9740265123469552533 ) ) ;
#2923=AXIS2_PLACEMENT_3D ( 'NONE', #2714, #7158, #3200 ) ;
#2939=FILL_AREA_STYLE_COLOUR ( '', #7001 ) ;
#2954=EDGE_LOOP ( 'NONE', ( #2251, #851, #4981, #1306 ) ) ;
#2967=DIRECTION ( 'NONE',  ( 0.9986925448795958005, 0.05111947575940636868, 5.682652305653510796E-17 ) ) ;
#2969=CARTESIAN_POINT ( 'NONE',  ( 27.99155020439386732, -34.64269665048638558, 3.999999999999966249 ) ) ;
#2978=CARTESIAN_POINT ( 'NONE',  ( 18.06432739836606416, -39.71205113188410252, -3.955074325938786408E-14 ) ) ;
#2986=ORIENTED_EDGE ( 'NONE', *, *, #253, .F. ) ;
#2989=CARTESIAN_POINT ( 'NONE',  ( 27.08917575328167615, -34.57010104422300145, -0.4368814963732711165 ) ) ;
#3018=ORIENTED_EDGE ( 'NONE', *, *, #393, .T. ) ;
#3051=CARTESIAN_POINT ( 'NONE',  ( 26.98506241315388010, -34.62942011279275079, -0.5000000000000346390 ) ) ;
#3055=CARTESIAN_POINT ( 'NONE',  ( 17.88843813672055916, -40.41242482140538073, -4.025211077939830175E-14 ) ) ;
#3062=ORIENTED_EDGE ( 'NONE', *, *, #2466, .T. ) ;
#3070=DIRECTION ( 'NONE',  ( 5.715354789845005112E-18, 9.999836672264339449E-16, -1.000000000000000000 ) ) ;
#3110=PLANE ( 'NONE',  #1847 ) ;
#3113=DIRECTION ( 'NONE',  ( 0.8688689365825388311, 0.4950421911735690128, -8.411011176753756085E-16 ) ) ;
#3119=DIRECTION ( 'NONE',  ( 5.715354789845004342E-18, 9.999836672264337477E-16, -1.000000000000000000 ) ) ;
#3128=AXIS2_PLACEMENT_3D ( 'NONE', #318, #7233, #2576 ) ;
#3129=PRODUCT_DEFINITION_SHAPE ( 'NONE', 'NONE',  #4117 ) ;
#3135=ORIENTED_EDGE ( 'NONE', *, *, #2818, .T. ) ;
#3137=ORIENTED_EDGE ( 'NONE', *, *, #235, .F. ) ;
#3160=AXIS2_PLACEMENT_3D ( 'NONE', #6265, #6342, #52 ) ;
#3170=ORIENTED_EDGE ( 'NONE', *, *, #2455, .T. ) ;
#3178=ORIENTED_EDGE ( 'NONE', *, *, #6154, .T. ) ;
#3180=EDGE_CURVE ( 'NONE', #2064, #7211, #7015, .T. ) ;
#3188=EDGE_CURVE ( 'NONE', #2830, #7250, #2237, .T. ) ;
#3198=FACE_OUTER_BOUND ( 'NONE', #3269, .T. ) ;
#3200=DIRECTION ( 'NONE',  ( -0.4950421911735689018, 0.8688689365825386091, 0.000000000000000000 ) ) ;
#3208=ORIENTED_EDGE ( 'NONE', *, *, #4353, .F. ) ;
#3221=DIRECTION ( 'NONE',  ( 0.4950421911735688463, -0.8688689365825387201, -8.660254037844397269E-16 ) ) ;
#3223=ORIENTED_EDGE ( 'NONE', *, *, #2455, .F. ) ;
#3236=ADVANCED_FACE ( 'NONE', ( #4225 ), #202, .T. ) ;
#3251=ORIENTED_EDGE ( 'NONE', *, *, #2818, .F. ) ;
#3252=ORIENTED_EDGE ( 'NONE', *, *, #5690, .F. ) ;
#3269=EDGE_LOOP ( 'NONE', ( #6616, #6172, #4347, #7146 ) ) ;
#3283=ADVANCED_FACE ( 'NONE', ( #93 ), #6522, .F. ) ;
#3284=ADVANCED_FACE ( 'NONE', ( #1917 ), #2386, .T. ) ;
#3327=CARTESIAN_POINT ( 'NONE',  ( 18.06432739836605350, -39.71205113188411673, -0.1321155921049125825 ) ) ;
#3334=DIRECTION ( 'NONE',  ( -0.4950421911735689018, 0.8688689365825386091, 0.000000000000000000 ) ) ;
#3336=EDGE_CURVE ( 'NONE', #1231, #6822, #4974, .T. ) ;
#3348=FACE_OUTER_BOUND ( 'NONE', #2631, .T. ) ;
#3371=DIRECTION ( 'NONE',  ( 5.715354789845005112E-18, 9.999836672264339449E-16, -1.000000000000000000 ) ) ;
#3374=CARTESIAN_POINT ( 'NONE',  ( 27.30483170388682623, -34.44723004512029974, -3.426145681764390930E-14 ) ) ;
#3388=AXIS2_PLACEMENT_3D ( 'NONE', #818, #3113, #3334 ) ;
#3390=CARTESIAN_POINT ( 'NONE',  ( 26.87807528571524074, -34.69037653529182563, 2.999999999999965361 ) ) ;
#3398=CARTESIAN_POINT ( 'NONE',  ( 18.63335487545880653, -39.96655599946684845, 3.999999999999960032 ) ) ;
#3406=CARTESIAN_POINT ( 'NONE',  ( 18.31184849395311787, -40.14648560017523238, 2.999999999999960032 ) ) ;
#3420=CIRCLE ( 'NONE', #1744, 140.0000000000000000 ) ;
#3430=CARTESIAN_POINT ( 'NONE',  ( 17.99698676687863852, -40.34744519239936267, 3.503909830570486328 ) ) ;
#3452=CARTESIAN_POINT ( 'NONE',  ( 27.13735696382475027, -34.54264957135247016, -0.3997825902234797835 ) ) ;
#3463=ORIENTED_EDGE ( 'NONE', *, *, #5743, .F. ) ;
#3464=CARTESIAN_POINT ( 'NONE',  ( 18.52223854178785345, -40.03305638412986411, 3.974049037550727803 ) ) ;
#3469=ORIENTED_EDGE ( 'NONE', *, *, #7135, .T. ) ;
#3477=CARTESIAN_POINT ( 'NONE',  ( 27.08917652808902687, -34.57010060277283969, 3.436818098114547748 ) ) ;
#3479=EDGE_LOOP ( 'NONE', ( #3931, #5729, #3252, #2034 ) ) ;
#3485=CARTESIAN_POINT ( 'NONE',  ( 27.40755238667390614, -34.38870444966534734, -0.8044411694303389426 ) ) ;
#3499=FACE_OUTER_BOUND ( 'NONE', #5471, .T. ) ;
#3504=EDGE_CURVE ( 'NONE', #936, #4310, #5830, .T. ) ;
#3511=CARTESIAN_POINT ( 'NONE',  ( 41.70778007397900211, -94.98992620957551480, 3.999999999999905409 ) ) ;
#3512=VECTOR ( 'NONE', #6155, 1000.000000000000000 ) ;
#3544=DIRECTION ( 'NONE',  ( -0.9999836672264333925, 0.005715354789844971292, -3.141587852546554631E-32 ) ) ;
#3549=CARTESIAN_POINT ( 'NONE',  ( 18.21884925479887940, -40.21464179917847304, -0.7992328572925022634 ) ) ;
#3562=CARTESIAN_POINT ( 'NONE',  ( 27.74785688037308518, -34.19481435285785409, -4.220975948576798359E-14 ) ) ;
#3581=CARTESIAN_POINT ( 'NONE',  ( 18.31450470689560461, -40.15738718825951992, -0.8737133221916458803 ) ) ;
#3586=VERTEX_POINT ( 'NONE', #5778 ) ;
#3592=DIRECTION ( 'NONE',  ( -0.9999836672264333925, 0.005715354789845005987, 4.554564057672517313E-33 ) ) ;
#3594=DIRECTION ( 'NONE',  ( -5.715354789845005112E-18, -9.999836672264339449E-16, 1.000000000000000000 ) ) ;
#3597=DIRECTION ( 'NONE',  ( 0.000000000000000000, 0.000000000000000000, 1.000000000000000000 ) ) ;
#3604=EDGE_CURVE ( 'NONE', #2388, #7211, #5953, .T. ) ;
#3615=CLOSED_SHELL ( 'NONE', ( #5776, #2777, #6140, #3640, #1321, #7424, #3899, #1681, #2357, #3792, #2087, #3944, #2086, #7095, #5267, #4112, #3283, #6741, #3284, #2635, #3236, #2194, #6936, #4030, #7000, #706 ) ) ;
#3617=CARTESIAN_POINT ( 'NONE',  ( 18.52082317230821928, -40.03390347989001441, -0.9734914404586040293 ) ) ;
#3627=( GEOMETRIC_REPRESENTATION_CONTEXT ( 3 ) GLOBAL_UNCERTAINTY_ASSIGNED_CONTEXT ( ( #2678 ) ) GLOBAL_UNIT_ASSIGNED_CONTEXT ( ( #2346, #4654, #2377 ) ) REPRESENTATION_CONTEXT ( 'NONE', 'WORKASPACE' ) );
#3628=AXIS2_PLACEMENT_3D ( 'NONE', #3406, #1159, #6916 ) ;
#3638=( NAMED_UNIT ( * ) SI_UNIT ( $, .STERADIAN. ) SOLID_ANGLE_UNIT ( ) );
#3640=ADVANCED_FACE ( 'NONE', ( #4107 ), #1074, .T. ) ;
#3652=EDGE_CURVE ( 'NONE', #6398, #2388, #6721, .T. ) ;
#3654=DIRECTION ( 'NONE',  ( 5.715354789845005112E-18, 9.999836672264339449E-16, -1.000000000000000000 ) ) ;
#3661=CARTESIAN_POINT ( 'NONE',  ( 18.07563673267965854, -39.70560758510323041, -0.1308779909158750421 ) ) ;
#3675=CARTESIAN_POINT ( 'NONE',  ( -105.7473861751082040, -118.0666774205683822, -1.186117176699141851E-13 ) ) ;
#3689=CARTESIAN_POINT ( 'NONE',  ( 18.44199058758350063, -39.49687574139178992, -0.4999999711863141738 ) ) ;
#3713=CARTESIAN_POINT ( 'NONE',  ( 43.95483829995806957, -94.87490738911687060, 3.999999999999905409 ) ) ;
#3719=EDGE_LOOP ( 'NONE', ( #5944, #4813, #4631, #1024, #546, #6420, #7201, #6153 ) ) ;
#3720=CARTESIAN_POINT ( 'NONE',  ( 43.95483829995806957, -94.87490738911687060, 3.999999999999905409 ) ) ;
#3725=CARTESIAN_POINT ( 'NONE',  ( 38.49686355599224896, -95.49243502991532750, 2.999999999999904521 ) ) ;
#3736=VECTOR ( 'NONE', #6161, 1000.000000000000000 ) ;
#3754=AXIS2_PLACEMENT_3D ( 'NONE', #6247, #3371, #5124 ) ;
#3757=ORIENTED_EDGE ( 'NONE', *, *, #6221, .F. ) ;
#3759=CARTESIAN_POINT ( 'NONE',  ( 43.95483829995806957, -94.87490738911687060, 2.999999999999905409 ) ) ;
#3769=DIRECTION ( 'NONE',  ( 5.715354789845005112E-18, 9.999836672264339449E-16, -1.000000000000000000 ) ) ;
#3775=AXIS2_PLACEMENT_3D ( 'NONE', #3675, #896, #6545 ) ;
#3782=VERTEX_POINT ( 'NONE', #3759 ) ;
#3792=ADVANCED_FACE ( 'NONE', ( #4262 ), #3829, .F. ) ;
#3800=FACE_OUTER_BOUND ( 'NONE', #6044, .T. ) ;
#3814=EDGE_LOOP ( 'NONE', ( #5910, #1101, #6448, #1596 ) ) ;
#3820=CARTESIAN_POINT ( 'NONE',  ( -95.86211798318534250, -102.0316339954322018, -1.000000000000102807 ) ) ;
#3825=CARTESIAN_POINT ( 'NONE',  ( 27.25760507213267658, -34.47413764220541310, -0.2615252949604586208 ) ) ;
#3829=CYLINDRICAL_SURFACE ( 'NONE', #6138, 140.0000000000000000 ) ;
#3842=DIRECTION ( 'NONE',  ( -7.159176919053500386E-18, -9.973300763855708376E-16, 1.000000000000000000 ) ) ;
#3844=LINE ( 'NONE', #5024, #3736 ) ;
#3863=DIRECTION ( 'NONE',  ( -0.9999836672264335036, 0.005715354789845008589, 0.000000000000000000 ) ) ;
#3868=CYLINDRICAL_SURFACE ( 'NONE', #4936, 0.4999999999999978906 ) ;
#3876=CARTESIAN_POINT ( 'NONE',  ( 17.61082880304171994, -39.97043410412675968, 2.999999999999957812 ) ) ;
#3883=DIRECTION ( 'NONE',  ( 0.000000000000000000, -1.000000000000000000, -8.673617379884027583E-16 ) ) ;
#3894=CARTESIAN_POINT ( 'NONE',  ( 27.29354050645795482, -34.45366325832522136, 3.130828461196526469 ) ) ;
#3899=ADVANCED_FACE ( 'NONE', ( #3348 ), #234, .T. ) ;
#3904=FACE_BOUND ( 'NONE', #4666, .T. ) ;
#3910=ORIENTED_EDGE ( 'NONE', *, *, #4724, .F. ) ;
#3912=( BOUNDED_SURFACE ( )  B_SPLINE_SURFACE ( 3, 2, ( 
 ( #72, #5764, #1727 ),
 ( #5163, #4026, #2283 ),
 ( #4134, #4672, #2921 ),
 ( #2989, #4703, #1168 ),
 ( #3452, #3485, #1798 ),
 ( #5273, #2393, #5804 ),
 ( #592, #30, #631 ),
 ( #2326, #5240, #2363 ),
 ( #6954, #7031, #6435 ),
 ( #1283, #3562, #136 ) ),
 .UNSPECIFIED., .F., .F., .T. ) 
 B_SPLINE_SURFACE_WITH_KNOTS ( ( 4, 2, 2, 2, 4 ),
 ( 3, 3 ),
 ( 0.000000000000000000, 0.0001952887240141836802, 0.0003905774480283673604, 0.0005858661720425509863, 0.0007811548960567347207 ),
 ( 0.000000000000000000, 1.000000000000000000 ),
 .UNSPECIFIED. ) 
 GEOMETRIC_REPRESENTATION_ITEM ( )  RATIONAL_B_SPLINE_SURFACE ( (
 ( 1.000000000000000000, 0.7071067811865472397, 1.000000000000000000),
 ( 1.000000000000000000, 0.7061982418737673406, 1.000000000000000000),
 ( 1.000000000000000000, 0.7052889306346207254, 1.000000000000000000),
 ( 1.000000000000000000, 0.7036054371094994098, 1.000000000000000000),
 ( 1.000000000000000000, 0.7028338995551517421, 1.000000000000000000),
 ( 1.000000000000000000, 0.7015497601672633365, 1.000000000000000000),
 ( 1.000000000000000000, 0.7010307650890416076, 1.000000000000000000),
 ( 1.000000000000000000, 0.7003352509067762854, 1.000000000000000000),
 ( 1.000000000000000000, 0.7001488311338350812, 1.000000000000000000),
 ( 1.000000000000000000, 0.7001503461741274137, 1.000000000000000000) ) ) 
 REPRESENTATION_ITEM ( '' )  SURFACE ( )  );
#3917=CARTESIAN_POINT ( 'NONE',  ( 17.88843813672056626, -40.41242482140539494, 2.999999999999957367 ) ) ;
#3928=CARTESIAN_POINT ( 'NONE',  ( 26.87031364676134970, -34.69479876584121314, 3.499999999999965805 ) ) ;
#3931=ORIENTED_EDGE ( 'NONE', *, *, #803, .F. ) ;
#3939=B_SPLINE_CURVE_WITH_KNOTS ( 'NONE', 3,
 ( #5751, #4832, #5863, #4691, #4158, #5368 ),
 .UNSPECIFIED., .F., .F.,
 ( 4, 2, 4 ),
 ( 0.000000000000000000, 0.0003937726336352555625, 0.0007875452672705111250 ),
 .UNSPECIFIED. ) ;
#3944=ADVANCED_FACE ( 'NONE', ( #6188 ), #4529, .T. ) ;
#3971=ORIENTED_EDGE ( 'NONE', *, *, #2036, .F. ) ;
#3974=EDGE_CURVE ( 'NONE', #6398, #5434, #6402, .T. ) ;
#3990=FACE_OUTER_BOUND ( 'NONE', #2741, .T. ) ;
#3996=CARTESIAN_POINT ( 'NONE',  ( 17.72543015532271937, -39.90513944096638710, 3.513721684389295330 ) ) ;
#4005=CARTESIAN_POINT ( 'NONE',  ( 17.88843813672054850, -40.41242482140538073, 3.264142021185714171 ) ) ;
#4007=AXIS2_PLACEMENT_3D ( 'NONE', #3511, #5225, #61 ) ;
#4008=AXIS2_PLACEMENT_3D ( 'NONE', #2877, #2841, #2804 ) ;
#4013=CARTESIAN_POINT ( 'NONE',  ( 27.24996190780300509, -34.47849237127667266, 3.251881639501436272 ) ) ;
#4019=ORIENTED_EDGE ( 'NONE', *, *, #7011, .T. ) ;
#4020=AXIS2_PLACEMENT_3D ( 'NONE', #387, #3594, #4387 ) ;
#4026=CARTESIAN_POINT ( 'NONE',  ( 26.98408672118752349, -34.62997601791116153, -1.001286369213168825 ) ) ;
#4030=ADVANCED_FACE ( 'NONE', ( #3990 ), #3868, .T. ) ;
#4041=CARTESIAN_POINT ( 'NONE',  ( 18.21934571153571980, -40.21434464133486841, 3.799679232396574236 ) ) ;
#4052=CARTESIAN_POINT ( 'NONE',  ( 27.09963614945447219, -34.56414118396787671, 3.975998075095239503 ) ) ;
#4071=ORIENTED_EDGE ( 'NONE', *, *, #6599, .F. ) ;
#4074=DIRECTION ( 'NONE',  ( 0.05111947575940102573, -0.9986925448795961335, 1.285697817222219874E-14 ) ) ;
#4077=CARTESIAN_POINT ( 'NONE',  ( 17.88843813672055916, -40.41242482140538783, 2.999999999999959588 ) ) ;
#4088=AXIS2_PLACEMENT_3D ( 'NONE', #1177, #5658, #5135 ) ;
#4107=FACE_OUTER_BOUND ( 'NONE', #3814, .T. ) ;
#4112=ADVANCED_FACE ( 'NONE', ( #4649 ), #5964, .T. ) ;
#4114=AXIS2_PLACEMENT_3D ( 'NONE', #6569, #5985, #4843 ) ;
#4117=PRODUCT_DEFINITION ( 'UNKNOWN', '', #6650, #2604 ) ;
#4119=AXIS2_PLACEMENT_3D ( 'NONE', #2891, #1778, #5213 ) ;
#4131=AXIS2_PLACEMENT_3D ( 'NONE', #7217, #2550, #4213 ) ;
#4134=CARTESIAN_POINT ( 'NONE',  ( 26.98398549905668986, -34.63003368969938123, -0.4870132424029344209 ) ) ;
#4157=DIRECTION ( 'NONE',  ( -0.4950421911735689018, 0.8688689365825386091, 0.000000000000000000 ) ) ;
#4158=CARTESIAN_POINT ( 'NONE',  ( 27.30483170388658820, -34.44723004512044184, 3.132067106505118215 ) ) ;
#4160=CARTESIAN_POINT ( 'NONE',  ( 17.95758103425560748, -39.77287037833651340, -0.8100516860784414686 ) ) ;
#4165=VERTEX_POINT ( 'NONE', #3725 ) ;
#4182=ORIENTED_EDGE ( 'NONE', *, *, #6829, .T. ) ;
#4195=EDGE_LOOP ( 'NONE', ( #4553, #4490, #3170, #5481 ) ) ;
#4203=CYLINDRICAL_SURFACE ( 'NONE', #767, 0.5000000000000004441 ) ;
#4213=DIRECTION ( 'NONE',  ( -0.9999836672264332815, 0.005715354789842956411, 0.000000000000000000 ) ) ;
#4219=FILL_AREA_STYLE ('',( #2939 ) ) ;
#4224=DIRECTION ( 'NONE',  ( -0.9999836672264333925, 0.005715354789844476896, 0.000000000000000000 ) ) ;
#4225=FACE_OUTER_BOUND ( 'NONE', #1014, .T. ) ;
#4262=FACE_OUTER_BOUND ( 'NONE', #5768, .T. ) ;
#4267=ORIENTED_EDGE ( 'NONE', *, *, #7135, .F. ) ;
#4270=DIRECTION ( 'NONE',  ( 5.715354789845005112E-18, 9.999836672264339449E-16, -1.000000000000000000 ) ) ;
#4272=EDGE_CURVE ( 'NONE', #4165, #6113, #5782, .T. ) ;
#4289=CARTESIAN_POINT ( 'NONE',  ( 41.70778007397900211, -94.98992620957551480, 2.999999999999905409 ) ) ;
#4301=DIRECTION ( 'NONE',  ( 0.8688689365825388311, 0.4950421911735690128, 0.000000000000000000 ) ) ;
#4304=FACE_OUTER_BOUND ( 'NONE', #6191, .T. ) ;
#4310=VERTEX_POINT ( 'NONE', #2228 ) ;
#4337=DIRECTION ( 'NONE',  ( 5.715354789845005112E-18, 9.999836672264339449E-16, -1.000000000000000000 ) ) ;
#4347=ORIENTED_EDGE ( 'NONE', *, *, #3336, .F. ) ;
#4352=CARTESIAN_POINT ( 'NONE',  ( 18.47982041150265431, -39.47532202006953383, 2.999999999999960476 ) ) ;
#4353=EDGE_CURVE ( 'NONE', #2276, #888, #5556, .T. ) ;
#4358=ORIENTED_EDGE ( 'NONE', *, *, #7011, .F. ) ;
#4379=CIRCLE ( 'NONE', #5472, 0.5000000000000004441 ) ;
#4387=DIRECTION ( 'NONE',  ( -0.9999836672264335036, 0.005715354789845008589, 0.000000000000000000 ) ) ;
#4396=CARTESIAN_POINT ( 'NONE',  ( 27.30483170388657044, -34.44723004512044895, 2.999999999999965805 ) ) ;
#4406=DIRECTION ( 'NONE',  ( -5.715354789845133764E-18, -9.999836672264337477E-16, 1.000000000000000000 ) ) ;
#4420=DIRECTION ( 'NONE',  ( 0.8688689365825387201, 0.4950421911735688463, 4.999999999999993486E-16 ) ) ;
#4432=ORIENTED_EDGE ( 'NONE', *, *, #2905, .F. ) ;
#4452=CARTESIAN_POINT ( 'NONE',  ( 18.05682814888138665, -39.71632386479095089, 3.883467497571597704 ) ) ;
#4482=CARTESIAN_POINT ( 'NONE',  ( -95.86211798318534250, -102.0316339954322018, -1.025655255171287195E-13 ) ) ;
#4490=ORIENTED_EDGE ( 'NONE', *, *, #7227, .F. ) ;
#4496=CARTESIAN_POINT ( 'NONE',  ( 18.11932642638120328, -39.68071517522289327, 3.251954915088070663 ) ) ;
#4510=CARTESIAN_POINT ( 'NONE',  ( 18.47982041150265786, -39.47532202006954094, -0.5000000000000394129 ) ) ;
#4512=CARTESIAN_POINT ( 'NONE',  ( 26.98474422010017904, -34.62960140479226112, 4.001293834245286618 ) ) ;
#4514=( BOUNDED_SURFACE ( )  B_SPLINE_SURFACE ( 3, 2, ( 
 ( #344, #7417, #502 ),
 ( #1181, #6307, #4568 ),
 ( #1625, #7302, #3464 ),
 ( #6902, #4452, #1063 ),
 ( #462, #5098, #4041 ),
 ( #6856, #1027, #1700 ),
 ( #4496, #3996, #3430 ),
 ( #6341, #5056, #2742 ),
 ( #5707, #5742, #5172 ),
 ( #2226, #3876, #3917 ) ),
 .UNSPECIFIED., .F., .F., .F. ) 
 B_SPLINE_SURFACE_WITH_KNOTS ( ( 4, 2, 2, 2, 4 ),
 ( 3, 3 ),
 ( 0.000000000000000000, 0.0001953596913251163321, 0.0003907193826502326642, 0.0005860790739753490505, 0.0007814387653004653284 ),
 ( 0.000000000000000000, 1.000000000000000000 ),
 .UNSPECIFIED. ) 
 GEOMETRIC_REPRESENTATION_ITEM ( )  RATIONAL_B_SPLINE_SURFACE ( (
 ( 1.000000000000000000, 0.7071067811865465735, 1.000000000000000000),
 ( 1.000000000000000000, 0.7051297887126681818, 1.000000000000000000),
 ( 1.000000000000000000, 0.7031405235181358293, 1.000000000000000000),
 ( 1.000000000000000000, 0.6994400710090995510, 1.000000000000000000),
 ( 1.000000000000000000, 0.6977350462886972027, 1.000000000000000000),
 ( 1.000000000000000000, 0.6948874123953024950, 1.000000000000000000),
 ( 1.000000000000000000, 0.6937311395898003719, 1.000000000000000000),
 ( 1.000000000000000000, 0.6921794382103451104, 1.000000000000000000),
 ( 1.000000000000000000, 0.6917621249165484265, 1.000000000000000000),
 ( 1.000000000000000000, 0.6917656125192588323, 1.000000000000000000) ) ) 
 REPRESENTATION_ITEM ( '' )  SURFACE ( )  );
#4529=CYLINDRICAL_SURFACE ( 'NONE', #4088, 147.0000000000000000 ) ;
#4538=ORIENTED_EDGE ( 'NONE', *, *, #1818, .T. ) ;
#4546=CARTESIAN_POINT ( 'NONE',  ( 27.31013720395375799, -34.44420721133294450, 3.877994099121481852 ) ) ;
#4553=ORIENTED_EDGE ( 'NONE', *, *, #1501, .F. ) ;
#4554=DIRECTION ( 'NONE',  ( 0.000000000000000000, 1.000000000000000000, 1.734723475976805517E-15 ) ) ;
#4568=CARTESIAN_POINT ( 'NONE',  ( 18.63446967293817735, -39.96588886641734462, 3.999999999999968026 ) ) ;
#4575=CARTESIAN_POINT ( 'NONE',  ( 18.74668230531430169, -39.89873697698325117, 3.999999999999960032 ) ) ;
#4584=ORIENTED_EDGE ( 'NONE', *, *, #3504, .T. ) ;
#4604=CARTESIAN_POINT ( 'NONE',  ( 27.99155020439383890, -34.64269665048639979, 2.999999999999965805 ) ) ;
#4610=VECTOR ( 'NONE', #6287, 1000.000000000000000 ) ;
#4615=VECTOR ( 'NONE', #1443, 1000.000000000000000 ) ;
#4627=CARTESIAN_POINT ( 'NONE',  ( 26.87031364676134970, -34.69479876584121314, 3.999999999999965361 ) ) ;
#4631=ORIENTED_EDGE ( 'NONE', *, *, #6843, .T. ) ;
#4633=AXIS2_PLACEMENT_3D ( 'NONE', #2457, #7049, #6007 ) ;
#4634=AXIS2_PLACEMENT_3D ( 'NONE', #2304, #1786, #1189 ) ;
#4642=ORIENTED_EDGE ( 'NONE', *, *, #140, .T. ) ;
#4645=CARTESIAN_POINT ( 'NONE',  ( 41.70778007397900211, -94.98992620957551480, -9.475926987523308753E-14 ) ) ;
#4649=FACE_OUTER_BOUND ( 'NONE', #445, .T. ) ;
#4654=( NAMED_UNIT ( * ) PLANE_ANGLE_UNIT ( ) SI_UNIT ( $, .RADIAN. ) );
#4666=EDGE_LOOP ( 'NONE', ( #1312, #3251, #7220, #4822 ) ) ;
#4672=CARTESIAN_POINT ( 'NONE',  ( 27.09819939871877637, -34.56495977950342535, -0.9765397587610813446 ) ) ;
#4681=DIRECTION ( 'NONE',  ( 5.715354789845005112E-18, 9.999836672264339449E-16, -1.000000000000000000 ) ) ;
#4682=ORIENTED_EDGE ( 'NONE', *, *, #235, .T. ) ;
#4691=CARTESIAN_POINT ( 'NONE',  ( 27.25776622504945124, -34.47404582456791644, 3.261208021432587589 ) ) ;
#4697=ORIENTED_EDGE ( 'NONE', *, *, #6506, .T. ) ;
#4699=VECTOR ( 'NONE', #2107, 1000.000000000000000 ) ;
#4703=CARTESIAN_POINT ( 'NONE',  ( 27.31013562793543770, -34.44420810927673671, -0.8781215038714056398 ) ) ;
#4710=CARTESIAN_POINT ( 'NONE',  ( 17.88843813672055916, -40.41242482140538783, 2.999999999999959588 ) ) ;
#4724=EDGE_CURVE ( 'NONE', #936, #6398, #83, .T. ) ;
#4725=CARTESIAN_POINT ( 'NONE',  ( 18.23173688611030485, -39.61666878346903076, -0.3996164340295632611 ) ) ;
#4740=FACE_OUTER_BOUND ( 'NONE', #7139, .T. ) ;
#4758=CARTESIAN_POINT ( 'NONE',  ( 27.30483170388656333, -34.44723004512044895, -0.1320675480243696243 ) ) ;
#4775=DIRECTION ( 'NONE',  ( 5.715354789845005112E-18, 9.999836672264339449E-16, -1.000000000000000000 ) ) ;
#4780=SHAPE_REPRESENTATION_RELATIONSHIP ( 'NONE' , 'NONE' ,  #5284, #1803 ) ;
#4787=CARTESIAN_POINT ( 'NONE',  ( 27.30483170388682979, -34.44723004512030684, 2.999999999999965805 ) ) ;
#4798=CARTESIAN_POINT ( 'NONE',  ( 18.15155958994787611, -39.66235017763963810, -0.3073999163891736330 ) ) ;
#4801=FACE_OUTER_BOUND ( 'NONE', #2954, .T. ) ;
#4813=ORIENTED_EDGE ( 'NONE', *, *, #2036, .T. ) ;
#4822=ORIENTED_EDGE ( 'NONE', *, *, #676, .T. ) ;
#4829=ORIENTED_EDGE ( 'NONE', *, *, #6959, .T. ) ;
#4832=CARTESIAN_POINT ( 'NONE',  ( 26.98506203061672792, -34.62942033074510562, 3.499999999999965361 ) ) ;
#4834=CARTESIAN_POINT ( 'NONE',  ( 18.06060404229330985, -40.30936335904925727, -0.6147998435448814858 ) ) ;
#4843=DIRECTION ( 'NONE',  ( -0.005715354789845003385, -0.9999836672264335036, -1.000000000000000472E-15 ) ) ;
#4856=LINE ( 'NONE', #6693, #7385 ) ;
#4862=CIRCLE ( 'NONE', #4131, 3.250000000000000888 ) ;
#4864=EDGE_CURVE ( 'NONE', #2388, #2243, #1142, .T. ) ;
#4876=CARTESIAN_POINT ( 'NONE',  ( 26.87031364676133194, -34.69479876584122024, -0.5000000000000345279 ) ) ;
#4877=DIRECTION ( 'NONE',  ( -0.9999836672264335036, 0.005715354789845008589, 0.000000000000000000 ) ) ;
#4908=VERTEX_POINT ( 'NONE', #6170 ) ;
#4936=AXIS2_PLACEMENT_3D ( 'NONE', #1097, #7413, #5089 ) ;
#4973=CARTESIAN_POINT ( 'NONE',  ( -95.86211798318534250, -102.0316339954322018, -1.025655255171287195E-13 ) ) ;
#4974=CIRCLE ( 'NONE', #2923, 0.5000000000000022204 ) ;
#4981=ORIENTED_EDGE ( 'NONE', *, *, #3652, .T. ) ;
#4988=LINE ( 'NONE', #5493, #1140 ) ;
#4990=DIRECTION ( 'NONE',  ( 0.000000000000000000, -1.000000000000000000, -9.973300763855647239E-16 ) ) ;
#5012=CARTESIAN_POINT ( 'NONE',  ( 18.49916120972750377, -39.46430250869199341, -0.5000000000000393019 ) ) ;
#5024=CARTESIAN_POINT ( 'NONE',  ( -108.8601514936008385, -112.6033348200152915, 3.999999999999886313 ) ) ;
#5034=ORIENTED_EDGE ( 'NONE', *, *, #6959, .F. ) ;
#5040=CARTESIAN_POINT ( 'NONE',  ( 17.61001731287966265, -39.97089645448942719, 3.999999999999960032 ) ) ;
#5056=CARTESIAN_POINT ( 'NONE',  ( 17.63495400270750224, -39.95668865737157205, 3.269138726291231034 ) ) ;
#5069=CARTESIAN_POINT ( 'NONE',  ( 27.72483002872544944, -34.20793401062830696, 3.264201108005380547 ) ) ;
#5085=CARTESIAN_POINT ( 'NONE',  ( 18.47982041150265431, -39.47532202006953383, 2.999999999999960476 ) ) ;
#5086=AXIS2_PLACEMENT_3D ( 'NONE', #450, #2733, #6554 ) ;
#5089=DIRECTION ( 'NONE',  ( 0.4950421911735801705, -0.8688689365825322808, 0.000000000000000000 ) ) ;
#5098=CARTESIAN_POINT ( 'NONE',  ( 17.95809745115200684, -39.77257614736446811, 3.810493591301452820 ) ) ;
#5104=CARTESIAN_POINT ( 'NONE',  ( 27.55235279947361349, -34.38166451341173513, 2.999999999999965805 ) ) ;
#5115=CARTESIAN_POINT ( 'NONE',  ( 27.96884669319430827, -34.65534042161862516, 3.261656933814885306 ) ) ;
#5117=B_SPLINE_CURVE_WITH_KNOTS ( 'NONE', 3,
 ( #5123, #7435, #626, #5236, #6245, #69 ),
 .UNSPECIFIED., .F., .F.,
 ( 4, 2, 4 ),
 ( 0.000000000000000000, 0.0003939438732545951058, 0.0007878877465091902116 ),
 .UNSPECIFIED. ) ;
#5123=CARTESIAN_POINT ( 'NONE',  ( 18.06432739836606771, -39.71205113188410962, 2.999999999999960476 ) ) ;
#5124=DIRECTION ( 'NONE',  ( -0.9999836672264332815, 0.005715354789842956411, 0.000000000000000000 ) ) ;
#5134=CARTESIAN_POINT ( 'NONE',  ( 38.49686355599224896, -95.49243502991532750, -9.519295074422728931E-14 ) ) ;
#5135=DIRECTION ( 'NONE',  ( -0.9999836672264335036, 0.005715354789845041548, 0.000000000000000000 ) ) ;
#5149=CARTESIAN_POINT ( 'NONE',  ( 17.88843813672053429, -40.41242482140540204, -0.1320686260247052324 ) ) ;
#5152=CARTESIAN_POINT ( 'NONE',  ( 27.55792178321159014, -34.88417723535314252, 3.873636197071128606 ) ) ;
#5163=CARTESIAN_POINT ( 'NONE',  ( 26.92714173160467084, -34.66242069539057979, -0.4999999559301231411 ) ) ;
#5167=CARTESIAN_POINT ( 'NONE',  ( 27.89660656231303193, -34.69557212064219698, -0.5230190109555528100 ) ) ;
#5172=CARTESIAN_POINT ( 'NONE',  ( 17.88843813737523192, -40.41242482244771850, 3.131634423728840488 ) ) ;
#5186=CARTESIAN_POINT ( 'NONE',  ( 18.74668230531428748, -39.89873697698326538, -0.5000000000000397460 ) ) ;
#5203=CARTESIAN_POINT ( 'NONE',  ( 39.48483786921892857, -95.33781693134928048, -9.519295074422728931E-14 ) ) ;
#5209=ORIENTED_EDGE ( 'NONE', *, *, #7227, .T. ) ;
#5213=DIRECTION ( 'NONE',  ( -0.005715354789845003385, -0.9999836672264335036, -1.000000000000000472E-15 ) ) ;
#5214=VECTOR ( 'NONE', #6769, 1000.000000000000000 ) ;
#5225=DIRECTION ( 'NONE',  ( -5.715354789845005112E-18, -9.999836672264339449E-16, 1.000000000000000000 ) ) ;
#5236=CARTESIAN_POINT ( 'NONE',  ( 18.27210872828645094, -39.59366673520705859, 3.445918334850228693 ) ) ;
#5240=CARTESIAN_POINT ( 'NONE',  ( 27.72433805554270592, -34.20821431467933138, -0.2658584296617393372 ) ) ;
#5245=CARTESIAN_POINT ( 'NONE',  ( 27.11783474234811919, -35.12923323413248511, -1.000000000000035083 ) ) ;
#5249=DIRECTION ( 'NONE',  ( 0.05111947575940102573, -0.9986925448795961335, -9.983840675197624659E-16 ) ) ;
#5259=ORIENTED_EDGE ( 'NONE', *, *, #84, .T. ) ;
#5262=CARTESIAN_POINT ( 'NONE',  ( 17.63445134299215056, -39.95697505012468298, -0.2674678461753002279 ) ) ;
#5267=ADVANCED_FACE ( 'NONE', ( #4801 ), #6050, .T. ) ;
#5268=EDGE_LOOP ( 'NONE', ( #1565, #6832, #927, #6738, #5878 ) ) ;
#5273=CARTESIAN_POINT ( 'NONE',  ( 27.21752237596963298, -34.49697494815714549, -0.3076110668159389161 ) ) ;
#5275=ORIENTED_EDGE ( 'NONE', *, *, #5690, .T. ) ;
#5284=SHAPE_REPRESENTATION ( 'Vinyl Handle Grips', ( #751 ), #989 ) ;
#5317=DIRECTION ( 'NONE',  ( 5.715354789845005112E-18, 9.999836672264339449E-16, -1.000000000000000000 ) ) ;
#5326=CARTESIAN_POINT ( 'NONE',  ( 17.85753840846644636, -40.40533092278068494, -0.5000000000000403011 ) ) ;
#5368=CARTESIAN_POINT ( 'NONE',  ( 27.30483170388682979, -34.44723004512030684, 2.999999999999965805 ) ) ;
#5386=DIRECTION ( 'NONE',  ( -0.9999836672264335036, 0.005715354789845041548, 0.000000000000000000 ) ) ;
#5390=FACE_OUTER_BOUND ( 'NONE', #2203, .T. ) ;
#5398=CARTESIAN_POINT ( 'NONE',  ( 18.63383769599579054, -39.96626706310059518, -1.000000000000039746 ) ) ;
#5404=EDGE_LOOP ( 'NONE', ( #46, #7102, #3178, #3757 ) ) ;
#5408=AXIS2_PLACEMENT_3D ( 'NONE', #2220, #49, #5740 ) ;
#5434=VERTEX_POINT ( 'NONE', #6233 ) ;
#5444=CIRCLE ( 'NONE', #2670, 0.5000000000000022204 ) ;
#5445=ORIENTED_EDGE ( 'NONE', *, *, #5460, .T. ) ;
#5451=DIRECTION ( 'NONE',  ( 5.715354789845005112E-18, 9.999836672264339449E-16, -1.000000000000000000 ) ) ;
#5455=CIRCLE ( 'NONE', #3754, 3.250000000000000888 ) ;
#5456=ORIENTED_EDGE ( 'NONE', *, *, #676, .F. ) ;
#5459=EDGE_CURVE ( 'NONE', #6398, #5505, #765, .T. ) ;
#5460=EDGE_CURVE ( 'NONE', #4310, #1236, #4379, .T. ) ;
#5471=EDGE_LOOP ( 'NONE', ( #4358, #3208, #5034, #3223 ) ) ;
#5472=AXIS2_PLACEMENT_3D ( 'NONE', #466, #3842, #4990 ) ;
#5481=ORIENTED_EDGE ( 'NONE', *, *, #2167, .T. ) ;
#5493=CARTESIAN_POINT ( 'NONE',  ( 27.12559638130199247, -35.12481100358304076, -1.000000000000035083 ) ) ;
#5496=VERTEX_POINT ( 'NONE', #1629 ) ;
#5497=EDGE_LOOP ( 'NONE', ( #1816, #2252, #4267, #33 ) ) ;
#5505=VERTEX_POINT ( 'NONE', #5104 ) ;
#5514=DIRECTION ( 'NONE',  ( -5.715354789845005112E-18, -9.999836672264339449E-16, 1.000000000000000000 ) ) ;
#5556=LINE ( 'NONE', #6266, #4699 ) ;
#5566=CARTESIAN_POINT ( 'NONE',  ( 27.30483166554891739, -34.44723006696351320, 3.065403626746449728 ) ) ;
#5573=FACE_OUTER_BOUND ( 'NONE', #6439, .T. ) ;
#5580=CIRCLE ( 'NONE', #407, 147.0000000000000000 ) ;
#5581=CARTESIAN_POINT ( 'NONE',  ( 27.11783474234811564, -35.12923323413249221, -0.5000000000000350830 ) ) ;
#5587=CIRCLE ( 'NONE', #7014, 0.9999999999999994449 ) ;
#5625=B_SPLINE_CURVE_WITH_KNOTS ( 'NONE', 3,
 ( #6518, #4758, #3825, #2526, #3051, #4876 ),
 .UNSPECIFIED., .F., .F.,
 ( 4, 2, 4 ),
 ( 0.000000000000000000, 0.0003937823932578689420, 0.0007875647865157378840 ),
 .UNSPECIFIED. ) ;
#5629=CARTESIAN_POINT ( 'NONE',  ( 44.95353084483765826, -94.82378791335750634, -9.454242944073598665E-14 ) ) ;
#5641=DIRECTION ( 'NONE',  ( 0.8688689365825388311, 0.4950421911735690128, 0.000000000000000000 ) ) ;
#5648=ORIENTED_EDGE ( 'NONE', *, *, #7295, .F. ) ;
#5658=DIRECTION ( 'NONE',  ( 5.715354789845005112E-18, 9.999836672264339449E-16, -1.000000000000000000 ) ) ;
#5672=VECTOR ( 'NONE', #4681, 1000.000000000000000 ) ;
#5676=CARTESIAN_POINT ( 'NONE',  ( 27.23276465633407284, -35.06523870642838858, 3.999999999999965361 ) ) ;
#5684=ORIENTED_EDGE ( 'NONE', *, *, #7327, .T. ) ;
#5690=EDGE_CURVE ( 'NONE', #6854, #3586, #6908, .T. ) ;
#5707=CARTESIAN_POINT ( 'NONE',  ( 18.06432742338256148, -39.71205111763084972, 3.065817211669312314 ) ) ;
#5717=CARTESIAN_POINT ( 'NONE',  ( 17.99681370199822439, -40.34754878873740580, -0.5037687939243526980 ) ) ;
#5729=ORIENTED_EDGE ( 'NONE', *, *, #1901, .F. ) ;
#5736=CARTESIAN_POINT ( 'NONE',  ( 27.55794480445177541, -34.88416442371428161, -0.8737476923743859869 ) ) ;
#5740=DIRECTION ( 'NONE',  ( -0.9999836672264333925, 0.005715354789844971292, -3.141587852546554631E-32 ) ) ;
#5741=EDGE_CURVE ( 'NONE', #7211, #5434, #3420, .T. ) ;
#5742=CARTESIAN_POINT ( 'NONE',  ( 17.61082885536508158, -39.97043407431674922, 3.134598002289771923 ) ) ;
#5743=EDGE_CURVE ( 'NONE', #555, #1354, #2574, .T. ) ;
#5751=CARTESIAN_POINT ( 'NONE',  ( 26.87031364676134970, -34.69479876584121314, 3.499999999999965361 ) ) ;
#5764=CARTESIAN_POINT ( 'NONE',  ( 26.87031364676133194, -34.69479876584122024, -1.000000000000034861 ) ) ;
#5768=EDGE_LOOP ( 'NONE', ( #1768, #2610, #4829, #3135 ) ) ;
#5773=CARTESIAN_POINT ( 'NONE',  ( 27.11783474234813340, -35.12923323413248511, 3.999999999999965361 ) ) ;
#5776=ADVANCED_FACE ( 'NONE', ( #4304 ), #1885, .T. ) ;
#5778=CARTESIAN_POINT ( 'NONE',  ( 17.88843813672053074, -40.41242482140540204, -4.025211077939831437E-14 ) ) ;
#5782=CIRCLE ( 'NONE', #6972, 145.9999999999999716 ) ;
#5804=CARTESIAN_POINT ( 'NONE',  ( 27.81599406684724229, -34.74046346518214534, -0.6152221228502958716 ) ) ;
#5814=AXIS2_PLACEMENT_3D ( 'NONE', #2068, #4337, #2637 ) ;
#5815=AXIS2_PLACEMENT_3D ( 'NONE', #4482, #7329, #3863 ) ;
#5819=SURFACE_SIDE_STYLE ('',( #1359 ) ) ;
#5820=CIRCLE ( 'NONE', #1123, 141.0000000000000284 ) ;
#5830=CIRCLE ( 'NONE', #3160, 0.5000000000000004441 ) ;
#5843=TOROIDAL_SURFACE ( 'NONE', #2811, 2.249999999999964917, 1.000000000000000000 ) ;
#5846=EDGE_CURVE ( 'NONE', #1231, #420, #533, .T. ) ;
#5850=ORIENTED_EDGE ( 'NONE', *, *, #6829, .F. ) ;
#5858=PRESENTATION_STYLE_ASSIGNMENT (( #51 ) ) ;
#5863=CARTESIAN_POINT ( 'NONE',  ( 27.09755250833208606, -34.56532834836465895, 3.445680074011886251 ) ) ;
#5864=CARTESIAN_POINT ( 'NONE',  ( 18.38473276620558750, -39.52949865626803927, -0.4867457206136995285 ) ) ;
#5871=ORIENTED_EDGE ( 'NONE', *, *, #2466, .F. ) ;
#5878=ORIENTED_EDGE ( 'NONE', *, *, #7380, .F. ) ;
#5888=CARTESIAN_POINT ( 'NONE',  ( 44.95353084483765826, -94.82378791335750634, 2.999999999999905409 ) ) ;
#5896=CARTESIAN_POINT ( 'NONE',  ( 18.38461951018646445, -39.52956318442134886, -1.002819413936762105 ) ) ;
#5906=LINE ( 'NONE', #731, #2793 ) ;
#5908=DIRECTION ( 'NONE',  ( 0.000000000000000000, 1.000000000000000000, 1.734723475976805517E-15 ) ) ;
#5910=ORIENTED_EDGE ( 'NONE', *, *, #3652, .F. ) ;
#5915=CARTESIAN_POINT ( 'NONE',  ( 39.48483786921892857, -95.33781693134928048, -9.519295074422728931E-14 ) ) ;
#5918=CARTESIAN_POINT ( 'NONE',  ( 43.95483829995806957, -94.87490738911687060, -1.000000000000094591 ) ) ;
#5920=VERTEX_POINT ( 'NONE', #5134 ) ;
#5935=CARTESIAN_POINT ( 'NONE',  ( 17.72531364449922719, -39.90520582355987500, -0.5137159595961888758 ) ) ;
#5944=ORIENTED_EDGE ( 'NONE', *, *, #5846, .T. ) ;
#5949=CARTESIAN_POINT ( 'NONE',  ( 27.99155020439382469, -34.64269665048638558, -3.446982116472166490E-14 ) ) ;
#5951=CARTESIAN_POINT ( 'NONE',  ( 26.87031364676133194, -34.69479876584122024, -0.5000000000000345279 ) ) ;
#5953=CIRCLE ( 'NONE', #6904, 0.9999999999999994449 ) ;
#5959=CARTESIAN_POINT ( 'NONE',  ( 0.000000000000000000, 0.000000000000000000, 0.000000000000000000 ) ) ;
#5964=CYLINDRICAL_SURFACE ( 'NONE', #709, 3.250000000000000888 ) ;
#5967=DIRECTION ( 'NONE',  ( -0.9999836672264335036, 0.005715354789845041548, 0.000000000000000000 ) ) ;
#5970=DIRECTION ( 'NONE',  ( -0.9999836672264333925, 0.005715354789844970425, 0.000000000000000000 ) ) ;
#5977=CARTESIAN_POINT ( 'NONE',  ( 17.91075855300138997, -40.39906292810271538, -0.2617559932753710794 ) ) ;
#5985=DIRECTION ( 'NONE',  ( 5.715354789845004342E-18, 9.999836672264337477E-16, -1.000000000000000000 ) ) ;
#5991=( NAMED_UNIT ( * ) PLANE_ANGLE_UNIT ( ) SI_UNIT ( $, .RADIAN. ) );
#5993=DIRECTION ( 'NONE',  ( 5.715354789845005112E-18, 9.999836672264339449E-16, -1.000000000000000000 ) ) ;
#6003=EDGE_CURVE ( 'NONE', #1354, #5920, #1379, .T. ) ;
#6007=DIRECTION ( 'NONE',  ( 0.000000000000000000, -1.000000000000000000, -9.999836672264333533E-16 ) ) ;
#6040=CARTESIAN_POINT ( 'NONE',  ( -95.86211798318534250, -102.0316339954322018, 3.999999999999897859 ) ) ;
#6044=EDGE_LOOP ( 'NONE', ( #1002, #1197, #4182, #2626 ) ) ;
#6050=CYLINDRICAL_SURFACE ( 'NONE', #3128, 141.0000000000000284 ) ;
#6057=CIRCLE ( 'NONE', #3388, 0.5000000000000022204 ) ;
#6098=DIRECTION ( 'NONE',  ( -0.9999836672264335036, 0.005715354789845041548, 0.000000000000000000 ) ) ;
#6113=VERTEX_POINT ( 'NONE', #4710 ) ;
#6122=CARTESIAN_POINT ( 'NONE',  ( -105.7473861751082040, -118.0666774205683822, -1.000000000000118794 ) ) ;
#6133=CARTESIAN_POINT ( 'NONE',  ( 27.74785688037307096, -34.19481435285786830, 2.999999999999965805 ) ) ;
#6138=AXIS2_PLACEMENT_3D ( 'NONE', #6040, #941, #819 ) ;
#6140=ADVANCED_FACE ( 'NONE', ( #1534 ), #5843, .T. ) ;
#6141=DIRECTION ( 'NONE',  ( -0.9999836672264333925, 0.005715354789843017994, -1.984263399433601008E-30 ) ) ;
#6148=DIRECTION ( 'NONE',  ( 5.715354789845005112E-18, 9.999836672264339449E-16, -1.000000000000000000 ) ) ;
#6153=ORIENTED_EDGE ( 'NONE', *, *, #1539, .T. ) ;
#6154=EDGE_CURVE ( 'NONE', #3586, #5920, #298, .T. ) ;
#6155=DIRECTION ( 'NONE',  ( 5.715354789845005112E-18, 9.999836672264339449E-16, -1.000000000000000000 ) ) ;
#6161=DIRECTION ( 'NONE',  ( -0.8688689365825387201, -0.4950421911735688463, -4.999999999999993486E-16 ) ) ;
#6170=CARTESIAN_POINT ( 'NONE',  ( 27.11783474234811919, -35.12923323413248511, -1.000000000000035083 ) ) ;
#6172=ORIENTED_EDGE ( 'NONE', *, *, #140, .F. ) ;
#6181=TOROIDAL_SURFACE ( 'NONE', #1478, 147.0000000000000000, 1.000000000000000000 ) ;
#6188=FACE_OUTER_BOUND ( 'NONE', #2100, .T. ) ;
#6191=EDGE_LOOP ( 'NONE', ( #1, #4682, #5445, #1854 ) ) ;
#6208=CARTESIAN_POINT ( 'NONE',  ( 27.63607196376285913, -34.25850433845761245, 3.508149587753143894 ) ) ;
#6214=SHAPE_DEFINITION_REPRESENTATION ( #3129, #5284 ) ;
#6221=EDGE_CURVE ( 'NONE', #4165, #5920, #4856, .T. ) ;
#6222=CARTESIAN_POINT ( 'NONE',  ( 27.55235279947333993, -34.88166451341173513, 2.999999999999965361 ) ) ;
#6231=DIRECTION ( 'NONE',  ( -0.9999836672264333925, 0.005715354789844984303, 0.000000000000000000 ) ) ;
#6233=CARTESIAN_POINT ( 'NONE',  ( 27.11783474234813340, -35.12923323413248511, 3.999999999999965361 ) ) ;
#6241=CARTESIAN_POINT ( 'NONE',  ( 18.11147093304812827, -39.68519087974932802, -0.2612916689653262403 ) ) ;
#6245=CARTESIAN_POINT ( 'NONE',  ( 18.38437121370851202, -39.52970465251538457, 3.499999999999965805 ) ) ;
#6247=CARTESIAN_POINT ( 'NONE',  ( 41.70778007397900211, -94.98992620957551480, 2.999999999999905409 ) ) ;
#6251=CARTESIAN_POINT ( 'NONE',  ( 18.74668230531430169, -39.89873697698325117, 3.999999999999960032 ) ) ;
#6265=CARTESIAN_POINT ( 'NONE',  ( 27.55235279947335414, -34.88166451341171381, -3.471129529363089628E-14 ) ) ;
#6266=CARTESIAN_POINT ( 'NONE',  ( -109.1076725891878567, -112.1689003517234227, 2.999999999999887201 ) ) ;
#6276=DIRECTION ( 'NONE',  ( -0.8688689365825387201, -0.4950421911735688463, -4.999999999999993486E-16 ) ) ;
#6278=CARTESIAN_POINT ( 'NONE',  ( 26.92746976600782816, -34.66223379623596657, 3.499999971184567293 ) ) ;
#6287=DIRECTION ( 'NONE',  ( 5.715354789845084461E-18, 9.999836672264339449E-16, -1.000000000000000000 ) ) ;
#6289=ORIENTED_EDGE ( 'NONE', *, *, #6599, .T. ) ;
#6291=VECTOR ( 'NONE', #717, 1000.000000000000000 ) ;
#6302=VECTOR ( 'NONE', #6148, 1000.000000000000000 ) ;
#6307=CARTESIAN_POINT ( 'NONE',  ( 18.38526242690743118, -39.52919687957394501, 4.002803558047675736 ) ) ;
#6314=CARTESIAN_POINT ( 'NONE',  ( 17.91074121684488674, -40.39907330555904963, -0.2616656984610406522 ) ) ;
#6318=CARTESIAN_POINT ( 'NONE',  ( 27.11783474234813340, -35.12923323413248511, 3.999999999999965361 ) ) ;
#6322=VERTEX_POINT ( 'NONE', #7323 ) ;
#6324=CARTESIAN_POINT ( 'NONE',  ( 43.95483829995806957, -94.87490738911687060, -9.454242944073598665E-14 ) ) ;
#6331=ORIENTED_EDGE ( 'NONE', *, *, #451, .T. ) ;
#6332=CARTESIAN_POINT ( 'NONE',  ( 27.34642260356996246, -35.00195026692180988, -0.9740222605457664606 ) ) ;
#6336=CARTESIAN_POINT ( 'NONE',  ( 27.99155020439384955, -34.64269665048637137, 3.132057286715485667 ) ) ;
#6341=CARTESIAN_POINT ( 'NONE',  ( 18.07587756468298679, -39.70547036992888223, 3.131697286032659733 ) ) ;
#6342=DIRECTION ( 'NONE',  ( -7.159176919053500386E-18, -9.973300763855708376E-16, 1.000000000000000000 ) ) ;
#6352=CARTESIAN_POINT ( 'NONE',  ( 27.13760594192228481, -34.54250771490235650, 3.399562066569207897 ) ) ;
#6392=PRODUCT ( 'Vinyl Handle Grips', 'Vinyl Handle Grips', '', ( #1721 ) ) ;
#6398=VERTEX_POINT ( 'NONE', #6804 ) ;
#6402=B_SPLINE_CURVE_WITH_KNOTS ( 'NONE', 3,
 ( #4604, #6336, #6812, #1021, #1059, #1655, #2889, #5773 ),
 .UNSPECIFIED., .F., .F.,
 ( 4, 2, 2, 4 ),
 ( 4.336808689942017736E-18, 0.0003905499302250284256, 0.0007810998604500525144, 0.001562199720900107631 ),
 .UNSPECIFIED. ) ;
#6413=CARTESIAN_POINT ( 'NONE',  ( -95.86211798318534250, -102.0316339954322018, 2.999999999999897859 ) ) ;
#6420=ORIENTED_EDGE ( 'NONE', *, *, #802, .T. ) ;
#6422=CARTESIAN_POINT ( 'NONE',  ( 17.61082880304171994, -39.97043410412674547, -3.981171391688891273E-14 ) ) ;
#6435=CARTESIAN_POINT ( 'NONE',  ( 27.99155020466450949, -34.64269665098379392, -0.1315720824427292768 ) ) ;
#6439=EDGE_LOOP ( 'NONE', ( #2246, #1117, #1004, #2802 ) ) ;
#6443=CARTESIAN_POINT ( 'NONE',  ( 41.70778007397900211, -94.98992620957551480, 3.999999999999905409 ) ) ;
#6448=ORIENTED_EDGE ( 'NONE', *, *, #5741, .F. ) ;
#6452=CARTESIAN_POINT ( 'NONE',  ( 18.28020160475467293, -39.58905578051523122, -0.4368566607114584555 ) ) ;
#6467=DIRECTION ( 'NONE',  ( 1.000000000000000000, 0.000000000000000000, 0.000000000000000000 ) ) ;
#6470=DIRECTION ( 'NONE',  ( -0.1546180985661130547, 0.9879743132267154726, 9.870744795757317374E-16 ) ) ;
#6482=CARTESIAN_POINT ( 'NONE',  ( 17.79228376992792349, -39.86704927745797988, -0.6257137034768931461 ) ) ;
#6491=VERTEX_POINT ( 'NONE', #5915 ) ;
#6506=EDGE_CURVE ( 'NONE', #555, #2243, #5587, .T. ) ;
#6518=CARTESIAN_POINT ( 'NONE',  ( 27.30483170388656333, -34.44723004512044895, -3.427979277949995323E-14 ) ) ;
#6520=CIRCLE ( 'NONE', #4020, 140.0000000000000000 ) ;
#6522=CYLINDRICAL_SURFACE ( 'NONE', #1844, 145.9999999999999716 ) ;
#6539=AXIS2_PLACEMENT_3D ( 'NONE', #2684, #1032, #3883 ) ;
#6545=DIRECTION ( 'NONE',  ( -0.9999836672264333925, 0.005715354789844984303, 0.000000000000000000 ) ) ;
#6554=DIRECTION ( 'NONE',  ( -0.9999836672264333925, 0.005715354789844476896, 0.000000000000000000 ) ) ;
#6561=DIRECTION ( 'NONE',  ( 5.715354789845005112E-18, 9.999836672264339449E-16, -1.000000000000000000 ) ) ;
#6569=CARTESIAN_POINT ( 'NONE',  ( -105.7473861751082040, -118.0666774205683822, -1.186117176699141851E-13 ) ) ;
#6575=ORIENTED_EDGE ( 'NONE', *, *, #750, .F. ) ;
#6592=DIRECTION ( 'NONE',  ( 0.000000000000000000, 1.000000000000000000, 1.734723475976805517E-15 ) ) ;
#6599=EDGE_CURVE ( 'NONE', #5920, #2243, #4862, .T. ) ;
#6601=DIRECTION ( 'NONE',  ( 5.715354789845005112E-18, 9.999836672264339449E-16, -1.000000000000000000 ) ) ;
#6616=ORIENTED_EDGE ( 'NONE', *, *, #750, .T. ) ;
#6639=CIRCLE ( 'NONE', #3628, 0.5000000000000004441 ) ;
#6644=DIRECTION ( 'NONE',  ( 5.715354789845005112E-18, 9.999836672264339449E-16, -1.000000000000000000 ) ) ;
#6650=PRODUCT_DEFINITION_FORMATION_WITH_SPECIFIED_SOURCE ( 'ANY', '', #6392, .NOT_KNOWN. ) ;
#6653=DIRECTION ( 'NONE',  ( -0.9999836672264333925, 0.005715354789845005987, 4.554564057672517313E-33 ) ) ;
#6673=B_SPLINE_CURVE_WITH_KNOTS ( 'NONE', 3,
 ( #584, #515, #2754, #6241, #3327, #474 ),
 .UNSPECIFIED., .F., .F.,
 ( 4, 2, 4 ),
 ( 0.000000000000000000, 0.0003938972045929564408, 0.0007877944091859128816 ),
 .UNSPECIFIED. ) ;
#6675=CARTESIAN_POINT ( 'NONE',  ( -105.7473861751082040, -118.0666774205683822, 2.999999999999881428 ) ) ;
#6693=CARTESIAN_POINT ( 'NONE',  ( 38.49686355599224896, -95.49243502991532750, 3.999999999999904521 ) ) ;
#6721=CIRCLE ( 'NONE', #1081, 141.0000000000000284 ) ;
#6733=EDGE_CURVE ( 'NONE', #6854, #6928, #453, .T. ) ;
#6738=ORIENTED_EDGE ( 'NONE', *, *, #3504, .F. ) ;
#6741=ADVANCED_FACE ( 'NONE', ( #968, #3904 ), #2249, .F. ) ;
#6762=CARTESIAN_POINT ( 'NONE',  ( 18.06432739836633061, -39.71205113188396041, -3.955074325938771262E-14 ) ) ;
#6767=CARTESIAN_POINT ( 'NONE',  ( 26.87031364676134970, -34.69479876584121314, 3.499999999999965361 ) ) ;
#6769=DIRECTION ( 'NONE',  ( -0.8688689365825387201, -0.4950421911735688463, -4.999999999999992500E-16 ) ) ;
#6776=ORIENTED_EDGE ( 'NONE', *, *, #3974, .F. ) ;
#6791=CARTESIAN_POINT ( 'NONE',  ( 18.06051344111304857, -40.30941759226211474, -0.6146628003278669095 ) ) ;
#6799=ORIENTED_EDGE ( 'NONE', *, *, #6221, .T. ) ;
#6804=CARTESIAN_POINT ( 'NONE',  ( 27.99155020439383890, -34.64269665048639979, 2.999999999999965805 ) ) ;
#6808=ORIENTED_EDGE ( 'NONE', *, *, #7043, .F. ) ;
#6812=CARTESIAN_POINT ( 'NONE',  ( 27.96885038066250573, -34.65533836771933096, 3.261638044264441039 ) ) ;
#6822=VERTEX_POINT ( 'NONE', #6251 ) ;
#6828=CARTESIAN_POINT ( 'NONE',  ( 27.88122153832714645, -34.70413869602577961, 3.503763267581128549 ) ) ;
#6829=EDGE_CURVE ( 'NONE', #4908, #555, #2448, .T. ) ;
#6832=ORIENTED_EDGE ( 'NONE', *, *, #261, .F. ) ;
#6843=EDGE_CURVE ( 'NONE', #7068, #1236, #2663, .T. ) ;
#6854=VERTEX_POINT ( 'NONE', #6762 ) ;
#6856=CARTESIAN_POINT ( 'NONE',  ( 18.15174781562791395, -39.66224293516708599, 3.307682183023668454 ) ) ;
#6867=CARTESIAN_POINT ( 'NONE',  ( 27.40805635163918907, -34.38841731323995532, 3.804002023004813271 ) ) ;
#6871=EDGE_LOOP ( 'NONE', ( #3137, #372, #3910, #4584 ) ) ;
#6891=DIRECTION ( 'NONE',  ( 0.8688689365825387201, 0.4950421911735688463, 4.999999999999993486E-16 ) ) ;
#6901=VECTOR ( 'NONE', #4406, 1000.000000000000000 ) ;
#6902=CARTESIAN_POINT ( 'NONE',  ( 18.28020086966458990, -39.58905619933629083, 3.436919340399352318 ) ) ;
#6904=AXIS2_PLACEMENT_3D ( 'NONE', #1779, #4074, #463 ) ;
#6908=CIRCLE ( 'NONE', #4633, 0.5000000000000004441 ) ;
#6913=VECTOR ( 'NONE', #6891, 1000.000000000000000 ) ;
#6916=DIRECTION ( 'NONE',  ( 0.000000000000000000, -1.000000000000000000, -8.673617379884027583E-16 ) ) ;
#6928=VERTEX_POINT ( 'NONE', #673 ) ;
#6932=CARTESIAN_POINT ( 'NONE',  ( 43.95483829995806957, -94.87490738911687060, -9.454242944073598665E-14 ) ) ;
#6936=ADVANCED_FACE ( 'NONE', ( #1203 ), #3912, .T. ) ;
#6954=CARTESIAN_POINT ( 'NONE',  ( 27.30483167885241969, -34.44723005938377014, -0.06578604103650731449 ) ) ;
#6959=EDGE_CURVE ( 'NONE', #3782, #2276, #6520, .T. ) ;
#6967=PLANE ( 'NONE',  #4119 ) ;
#6972=AXIS2_PLACEMENT_3D ( 'NONE', #386, #1549, #6231 ) ;
#6981=B_SPLINE_CURVE_WITH_KNOTS ( 'NONE', 3,
 ( #60, #5149, #6314, #5717, #6791, #7426, #2866, #2268 ),
 .UNSPECIFIED., .F., .F.,
 ( 4, 2, 2, 4 ),
 ( 4.924395521842310123E-19, 0.0003905878508574884894, 0.0007811757017149765451, 0.001562351403429946151 ),
 .UNSPECIFIED. ) ;
#6993=CARTESIAN_POINT ( 'NONE',  ( 39.48483786921892857, -95.33781693134928048, 2.999999999999904521 ) ) ;
#7000=ADVANCED_FACE ( 'NONE', ( #349 ), #4203, .T. ) ;
#7001=COLOUR_RGB ( '', 0.09019608, 0.27058824, 0.51372549) ;
#7011=EDGE_CURVE ( 'NONE', #888, #1198, #169, .T. ) ;
#7014=AXIS2_PLACEMENT_3D ( 'NONE', #6932, #5249, #2967 ) ;
#7015=CIRCLE ( 'NONE', #4007, 2.249999999999962252 ) ;
#7031=CARTESIAN_POINT ( 'NONE',  ( 27.74785682929057629, -34.19481438196219614, -0.1328907850162961701 ) ) ;
#7043=EDGE_CURVE ( 'NONE', #5496, #4908, #4988, .T. ) ;
#7049=DIRECTION ( 'NONE',  ( -5.715354789851314459E-18, -9.999836672264284229E-16, 1.000000000000000000 ) ) ;
#7059=FACE_OUTER_BOUND ( 'NONE', #1131, .T. ) ;
#7068=VERTEX_POINT ( 'NONE', #4787 ) ;
#7081=CARTESIAN_POINT ( 'NONE',  ( 18.26921625715436193, -39.59531473433197135, -0.9790311301541629874 ) ) ;
#7086=ORIENTED_EDGE ( 'NONE', *, *, #1182, .F. ) ;
#7088=EDGE_CURVE ( 'NONE', #1354, #5496, #745, .T. ) ;
#7095=ADVANCED_FACE ( 'NONE', ( #5390 ), #3110, .F. ) ;
#7101=ORIENTED_EDGE ( 'NONE', *, *, #6506, .F. ) ;
#7102=ORIENTED_EDGE ( 'NONE', *, *, #2905, .T. ) ;
#7108=AXIS2_PLACEMENT_3D ( 'NONE', #6122, #3119, #2601 ) ;
#7117=PLANE ( 'NONE',  #7108 ) ;
#7119=CARTESIAN_POINT ( 'NONE',  ( 18.49916120972751088, -39.46430250869198630, -1.000000000000039524 ) ) ;
#7135=EDGE_CURVE ( 'NONE', #4165, #2064, #7375, .T. ) ;
#7139=EDGE_LOOP ( 'NONE', ( #7086, #4642, #460, #3469 ) ) ;
#7146=ORIENTED_EDGE ( 'NONE', *, *, #1539, .F. ) ;
#7148=CARTESIAN_POINT ( 'NONE',  ( -105.7473861751082040, -118.0666774205683822, 3.999999999999881428 ) ) ;
#7158=DIRECTION ( 'NONE',  ( 0.8688689365825388311, 0.4950421911735690128, -8.411011176753749182E-16 ) ) ;
#7168=DIRECTION ( 'NONE',  ( 5.715354789845005112E-18, 9.999836672264339449E-16, -1.000000000000000000 ) ) ;
#7201=ORIENTED_EDGE ( 'NONE', *, *, #6733, .T. ) ;
#7211=VERTEX_POINT ( 'NONE', #3713 ) ;
#7217=CARTESIAN_POINT ( 'NONE',  ( 41.70778007397900211, -94.98992620957551480, -9.475926987523308753E-14 ) ) ;
#7220=ORIENTED_EDGE ( 'NONE', *, *, #4353, .T. ) ;
#7227=EDGE_CURVE ( 'NONE', #1198, #6491, #7261, .T. ) ;
#7233=DIRECTION ( 'NONE',  ( 5.715354789845005112E-18, 9.999836672264339449E-16, -1.000000000000000000 ) ) ;
#7250=VERTEX_POINT ( 'NONE', #5012 ) ;
#7261=LINE ( 'NONE', #375, #6302 ) ;
#7275=CARTESIAN_POINT ( 'NONE',  ( -105.7473861751082040, -118.0666774205683822, -1.186117176699141851E-13 ) ) ;
#7295=EDGE_CURVE ( 'NONE', #2243, #936, #5820, .T. ) ;
#7302=CARTESIAN_POINT ( 'NONE',  ( 18.27066553070502408, -39.59448900386337300, 3.979556571570188162 ) ) ;
#7313=CARTESIAN_POINT ( 'NONE',  ( 27.34784330342383640, -35.00115915984075343, 3.973470358432956040 ) ) ;
#7323=CARTESIAN_POINT ( 'NONE',  ( 26.87807528571524074, -34.69037653529182563, -3.447762908503904100E-14 ) ) ;
#7327=EDGE_CURVE ( 'NONE', #6322, #2009, #939, .T. ) ;
#7329=DIRECTION ( 'NONE',  ( -5.715354789845005112E-18, -9.999836672264339449E-16, 1.000000000000000000 ) ) ;
#7351=CIRCLE ( 'NONE', #2177, 0.5000000000000004441 ) ;
#7352=CARTESIAN_POINT ( 'NONE',  ( 27.21771279145922406, -34.49686645803022600, 3.307326028875293478 ) ) ;
#7375=CIRCLE ( 'NONE', #4634, 1.000000000000001998 ) ;
#7379=AXIS2_PLACEMENT_3D ( 'NONE', #5203, #6470, #1316 ) ;
#7380=EDGE_CURVE ( 'NONE', #4908, #936, #556, .T. ) ;
#7385=VECTOR ( 'NONE', #932, 1000.000000000000000 ) ;
#7395=CARTESIAN_POINT ( 'NONE',  ( 27.81637696285268291, -34.74025023524533395, 3.614652068524565109 ) ) ;
#7403=CARTESIAN_POINT ( 'NONE',  ( 18.31184849395310721, -40.14648560017521106, 3.999999999999959144 ) ) ;
#7410=DIRECTION ( 'NONE',  ( 5.715354789845005112E-18, 9.999836672264339449E-16, -1.000000000000000000 ) ) ;
#7413=DIRECTION ( 'NONE',  ( -0.8688689365825387201, -0.4950421911735688463, -4.999999999999993486E-16 ) ) ;
#7417=CARTESIAN_POINT ( 'NONE',  ( 18.49916120972755351, -39.46430250869197209, 3.999999999999961808 ) ) ;
#7424=ADVANCED_FACE ( 'NONE', ( #1092 ), #637, .T. ) ;
#7426=CARTESIAN_POINT ( 'NONE',  ( 18.29784290781275757, -40.16735820407432556, -0.8913619061384294717 ) ) ;
#7435=CARTESIAN_POINT ( 'NONE',  ( 18.06432739836606771, -39.71205113188411673, 3.132117705585802270 ) ) ;
#7437=FACE_OUTER_BOUND ( 'NONE', #2847, .T. ) ;
ENDSEC;
END-ISO-10303-21;
